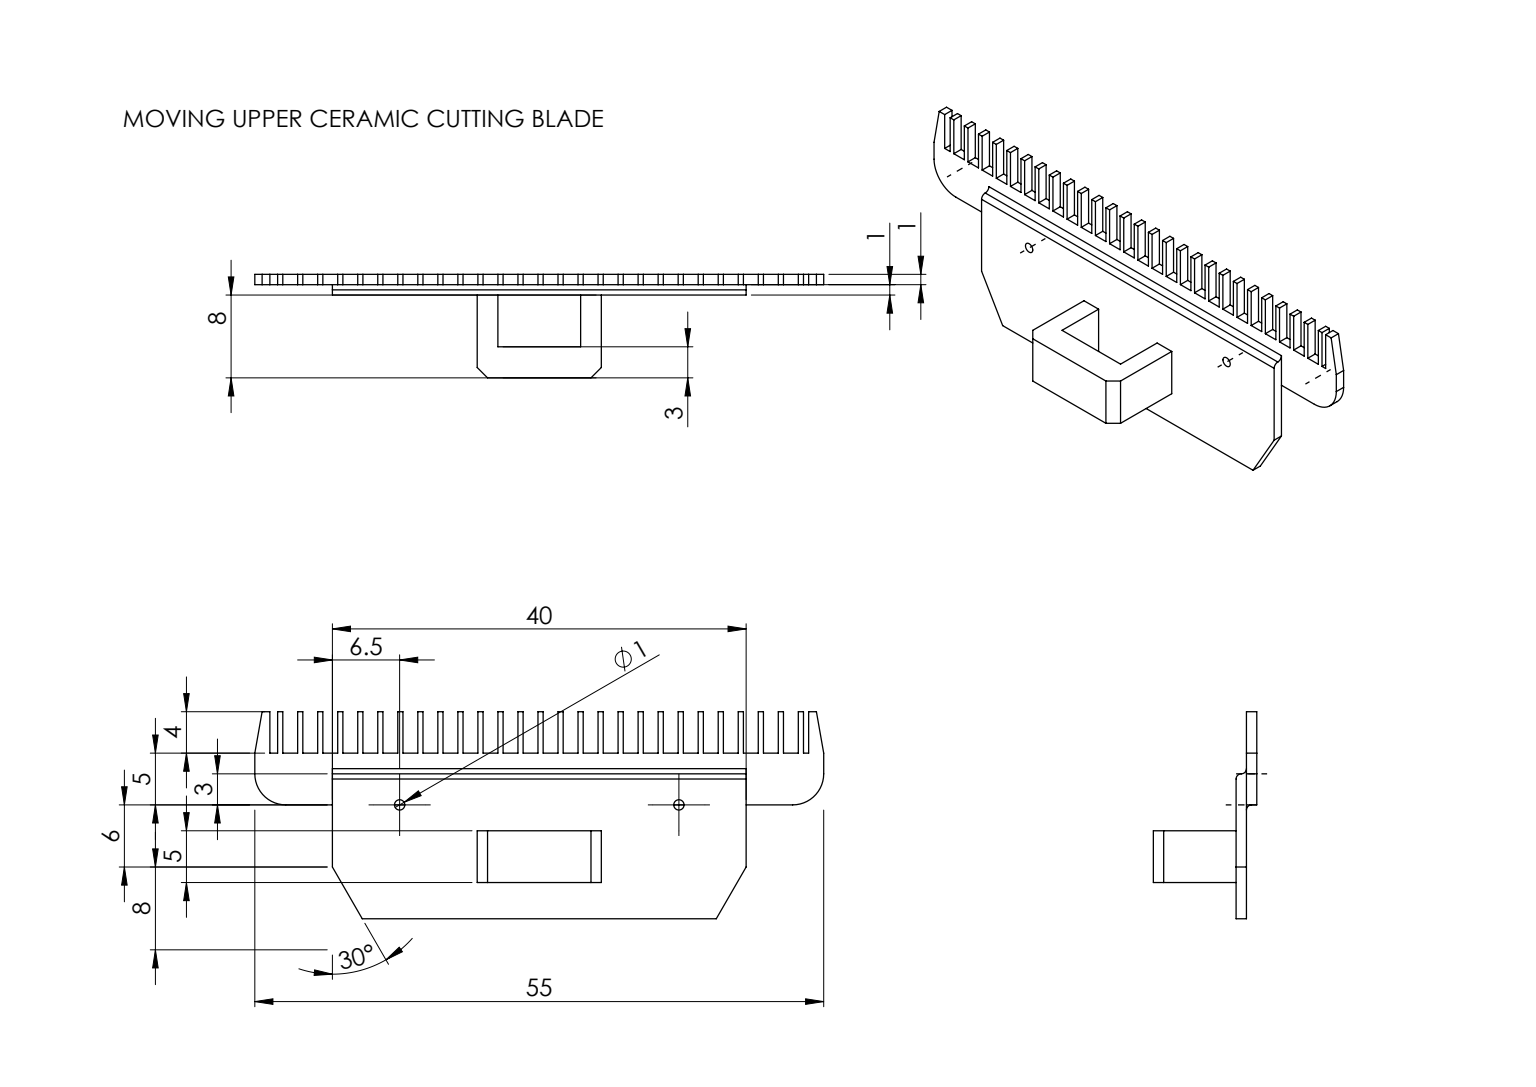
ISO-10303-21;
HEADER;
FILE_DESCRIPTION (('STEP AP214'),
    '1' );
FILE_NAME ('Moving Upper Ceramic Cutting Blade.step',
    '2026-10-04T16:38:04',
    ( '' ),
    ( '' ),
    'SwSTEP 2.0',
    'SolidWorks 2026',
    '' );
FILE_SCHEMA (( 'AUTOMOTIVE_DESIGN' ));
ENDSEC;

DATA;
#15=VECTOR ( 'NONE', #20550, 1000.000000000000000 ) ;
#17=VERTEX_POINT ( 'NONE', #19101 ) ;
#19=VERTEX_POINT ( 'NONE', #1418 ) ;
#21=FACE_BOUND ( 'NONE', #10951, .T. ) ;
#22=VECTOR ( 'NONE', #3512, 1000.000000000000000 ) ;
#26=FACE_OUTER_BOUND ( 'NONE', #4692, .T. ) ;
#35=ORIENTED_EDGE ( 'NONE', *, *, #2432, .F. ) ;
#42=VERTEX_POINT ( 'NONE', #6438 ) ;
#47=VECTOR ( 'NONE', #8617, 1000.000000000000000 ) ;
#49=VERTEX_POINT ( 'NONE', #11237 ) ;
#53=LINE ( 'NONE', #6129, #8350 ) ;
#54=AXIS2_PLACEMENT_3D ( 'NONE', #18555, #20450, #10501 ) ;
#56=LINE ( 'NONE', #9565, #7988 ) ;
#58=LINE ( 'NONE', #8001, #5190 ) ;
#60=CARTESIAN_POINT ( 'NONE',  ( 10.05565079891005631, 0.000000000000000000, 1.000000000000000000 ) ) ;
#61=LINE ( 'NONE', #4966, #6978 ) ;
#63=DIRECTION ( 'NONE',  ( 1.000000000000000000, 0.000000000000000000, 0.000000000000000000 ) ) ;
#68=VERTEX_POINT ( 'NONE', #1726 ) ;
#76=ORIENTED_EDGE ( 'NONE', *, *, #12428, .T. ) ;
#77=LINE ( 'NONE', #272, #14093 ) ;
#78=ORIENTED_EDGE ( 'NONE', *, *, #4872, .F. ) ;
#87=LINE ( 'NONE', #11371, #8961 ) ;
#89=( NAMED_UNIT ( * ) PLANE_ANGLE_UNIT ( ) SI_UNIT ( $, .RADIAN. ) );
#91=ORIENTED_EDGE ( 'NONE', *, *, #1253, .F. ) ;
#96=ADVANCED_FACE ( 'NONE', ( #6747 ), #14788, .T. ) ;
#98=DIRECTION ( 'NONE',  ( 0.000000000000000000, 1.000000000000000000, 0.000000000000000000 ) ) ;
#99=ORIENTED_EDGE ( 'NONE', *, *, #2749, .T. ) ;
#101=EDGE_LOOP ( 'NONE', ( #4164, #18704, #19121, #9760 ) ) ;
#102=VECTOR ( 'NONE', #3699, 1000.000000000000000 ) ;
#107=DIRECTION ( 'NONE',  ( -1.000000000000000000, 0.000000000000000000, 0.000000000000000000 ) ) ;
#114=VECTOR ( 'NONE', #15578, 1000.000000000000000 ) ;
#115=LINE ( 'NONE', #12457, #8728 ) ;
#121=ORIENTED_EDGE ( 'NONE', *, *, #545, .F. ) ;
#122=VERTEX_POINT ( 'NONE', #13311 ) ;
#126=ORIENTED_EDGE ( 'NONE', *, *, #7427, .F. ) ;
#128=CARTESIAN_POINT ( 'NONE',  ( 5.683390479346035029, 0.000000000000000000, 0.000000000000000000 ) ) ;
#134=CARTESIAN_POINT ( 'NONE',  ( -15.11404127825609223, 9.000000000000001776, 0.000000000000000000 ) ) ;
#137=LINE ( 'NONE', #12477, #19758 ) ;
#148=CARTESIAN_POINT ( 'NONE',  ( -24.79469207716615031, 9.000000000000001776, 1.000000000000000000 ) ) ;
#153=DIRECTION ( 'NONE',  ( 1.734723475976807094E-15, -1.000000000000000000, 0.000000000000000000 ) ) ;
#156=ORIENTED_EDGE ( 'NONE', *, *, #12533, .T. ) ;
#159=DIRECTION ( 'NONE',  ( 1.000000000000000000, 0.000000000000000000, 0.000000000000000000 ) ) ;
#161=CARTESIAN_POINT ( 'NONE',  ( 0.3749999999999968914, 9.000000000000000000, 1.000000000000000000 ) ) ;
#168=EDGE_LOOP ( 'NONE', ( #6512, #8849, #9507, #11718, #13942, #16405 ) ) ;
#170=DIRECTION ( 'NONE',  ( -0.000000000000000000, -0.000000000000000000, -1.000000000000000000 ) ) ;
#174=EDGE_CURVE ( 'NONE', #8535, #2052, #465, .T. ) ;
#177=ORIENTED_EDGE ( 'NONE', *, *, #14375, .F. ) ;
#179=FACE_OUTER_BOUND ( 'NONE', #19675, .T. ) ;
#180=AXIS2_PLACEMENT_3D ( 'NONE', #10679, #7642, #12344 ) ;
#187=LINE ( 'NONE', #10011, #17890 ) ;
#195=EDGE_CURVE ( 'NONE', #11770, #17871, #16650, .T. ) ;
#202=ORIENTED_EDGE ( 'NONE', *, *, #15005, .F. ) ;
#205=DIRECTION ( 'NONE',  ( 0.000000000000000000, -1.000000000000000000, 0.000000000000000000 ) ) ;
#208=DIRECTION ( 'NONE',  ( -0.9848077530122082424, 0.1736481776669295263, 0.000000000000000000 ) ) ;
#230=DIRECTION ( 'NONE',  ( -1.000000000000000000, -0.000000000000000000, -0.000000000000000000 ) ) ;
#231=CARTESIAN_POINT ( 'NONE',  ( 3.999999999999999112, -7.500000000000047073, 9.999999999999998224 ) ) ;
#259=EDGE_LOOP ( 'NONE', ( #9919, #6781, #19047, #17582 ) ) ;
#263=ORIENTED_EDGE ( 'NONE', *, *, #15990, .F. ) ;
#266=FACE_OUTER_BOUND ( 'NONE', #16647, .T. ) ;
#270=VECTOR ( 'NONE', #15636, 1000.000000000000000 ) ;
#272=CARTESIAN_POINT ( 'NONE',  ( 0.000000000000000000, 0.000000000000000000, 0.000000000000000000 ) ) ;
#274=ORIENTED_EDGE ( 'NONE', *, *, #17333, .T. ) ;
#278=LINE ( 'NONE', #14715, #12697 ) ;
#282=AXIS2_PLACEMENT_3D ( 'NONE', #5586, #11856, #17932 ) ;
#294=CARTESIAN_POINT ( 'NONE',  ( -3.497260319564023057, 9.000000000000001776, 0.000000000000000000 ) ) ;
#295=DIRECTION ( 'NONE',  ( 1.000000000000000000, 0.000000000000000000, 0.000000000000000000 ) ) ;
#302=VECTOR ( 'NONE', #7934, 1000.000000000000000 ) ;
#304=AXIS2_PLACEMENT_3D ( 'NONE', #2180, #611, #8776 ) ;
#305=ORIENTED_EDGE ( 'NONE', *, *, #7234, .F. ) ;
#306=VECTOR ( 'NONE', #18807, 1000.000000000000000 ) ;
#312=PLANE ( 'NONE',  #2667 ) ;
#324=ORIENTED_EDGE ( 'NONE', *, *, #17670, .T. ) ;
#325=ORIENTED_EDGE ( 'NONE', *, *, #12049, .T. ) ;
#328=CARTESIAN_POINT ( 'NONE',  ( 9.830951894845298966, -7.500000000000047073, 7.000000000000000000 ) ) ;
#331=EDGE_LOOP ( 'NONE', ( #16127, #14470, #13660, #8482 ) ) ;
#335=VECTOR ( 'NONE', #866, 1000.000000000000000 ) ;
#337=VECTOR ( 'NONE', #729, 1000.000000000000000 ) ;
#340=CARTESIAN_POINT ( 'NONE',  ( 0.000000000000000000, 4.999999999999999112, 1.000000000000000000 ) ) ;
#355=ORIENTED_EDGE ( 'NONE', *, *, #1510, .F. ) ;
#357=VECTOR ( 'NONE', #14447, 1000.000000000000000 ) ;
#358=ORIENTED_EDGE ( 'NONE', *, *, #6960, .T. ) ;
#360=CARTESIAN_POINT ( 'NONE',  ( 1.811130159782011528, 4.999999999999999112, 0.000000000000000000 ) ) ;
#366=CARTESIAN_POINT ( 'NONE',  ( 26.04469207716615031, 4.999999999999999112, 0.000000000000000000 ) ) ;
#367=VECTOR ( 'NONE', #7889, 1000.000000000000000 ) ;
#369=DIRECTION ( 'NONE',  ( -0.000000000000000000, 0.000000000000000000, -1.000000000000000000 ) ) ;
#370=DIRECTION ( 'NONE',  ( 0.000000000000000000, 1.000000000000000000, 0.000000000000000000 ) ) ;
#374=EDGE_LOOP ( 'NONE', ( #263, #11336, #20204, #3234 ) ) ;
#381=VERTEX_POINT ( 'NONE', #2855 ) ;
#385=ORIENTED_EDGE ( 'NONE', *, *, #8922, .T. ) ;
#404=DIRECTION ( 'NONE',  ( 1.000000000000000000, 0.000000000000000000, -0.000000000000000000 ) ) ;
#406=ORIENTED_EDGE ( 'NONE', *, *, #5858, .F. ) ;
#413=VECTOR ( 'NONE', #1830, 1000.000000000000000 ) ;
#416=DIRECTION ( 'NONE',  ( 0.000000000000000000, 1.000000000000000000, 0.000000000000000000 ) ) ;
#417=EDGE_CURVE ( 'NONE', #11328, #740, #20025, .T. ) ;
#427=VECTOR ( 'NONE', #3877, 1000.000000000000000 ) ;
#430=ORIENTED_EDGE ( 'NONE', *, *, #12679, .F. ) ;
#431=VERTEX_POINT ( 'NONE', #15503 ) ;
#435=ORIENTED_EDGE ( 'NONE', *, *, #9741, .F. ) ;
#448=EDGE_CURVE ( 'NONE', #18810, #17042, #19331, .T. ) ;
#457=CARTESIAN_POINT ( 'NONE',  ( -17.05017143803810242, 9.000000000000001776, 0.000000000000000000 ) ) ;
#458=VERTEX_POINT ( 'NONE', #10427 ) ;
#460=EDGE_LOOP ( 'NONE', ( #13036, #3328, #19557, #13078 ) ) ;
#463=DIRECTION ( 'NONE',  ( 0.000000000000000000, 1.000000000000000000, -0.000000000000000000 ) ) ;
#465=LINE ( 'NONE', #16554, #12981 ) ;
#469=LINE ( 'NONE', #14791, #1048 ) ;
#471=EDGE_CURVE ( 'NONE', #20320, #1300, #20347, .T. ) ;
#476=ORIENTED_EDGE ( 'NONE', *, *, #6440, .F. ) ;
#480=ORIENTED_EDGE ( 'NONE', *, *, #12324, .T. ) ;
#484=CARTESIAN_POINT ( 'NONE',  ( 0.000000000000000000, 9.000000000000001776, 1.000000000000000000 ) ) ;
#485=VERTEX_POINT ( 'NONE', #18066 ) ;
#487=VERTEX_POINT ( 'NONE', #8855 ) ;
#493=CARTESIAN_POINT ( 'NONE',  ( 3.999999999999999112, -2.500000000000047518, 7.000000000000000000 ) ) ;
#495=CARTESIAN_POINT ( 'NONE',  ( -11.24178095869206828, 0.000000000000000000, 1.000000000000000000 ) ) ;
#502=DIRECTION ( 'NONE',  ( -0.000000000000000000, -0.000000000000000000, -1.000000000000000000 ) ) ;
#504=ORIENTED_EDGE ( 'NONE', *, *, #11433, .F. ) ;
#506=ORIENTED_EDGE ( 'NONE', *, *, #871, .T. ) ;
#509=( GEOMETRIC_REPRESENTATION_CONTEXT ( 3 ) GLOBAL_UNCERTAINTY_ASSIGNED_CONTEXT ( ( #11112 ) ) GLOBAL_UNIT_ASSIGNED_CONTEXT ( ( #4790, #89, #18824 ) ) REPRESENTATION_CONTEXT ( 'NONE', 'WORKASPACE' ) );
#510=VERTEX_POINT ( 'NONE', #18268 ) ;
#511=DIRECTION ( 'NONE',  ( 0.000000000000000000, 1.000000000000000000, -0.000000000000000000 ) ) ;
#516=CARTESIAN_POINT ( 'NONE',  ( -13.50000000000000178, 0.000000000000000000, 2.000000000000000000 ) ) ;
#521=DIRECTION ( 'NONE',  ( 1.000000000000000000, 0.000000000000000000, 0.000000000000000000 ) ) ;
#537=SHAPE_REPRESENTATION ( 'Moving Upper Ceramic Cutting Blade', ( #18039 ), #19052 ) ;
#538=DIRECTION ( 'NONE',  ( -0.000000000000000000, -0.000000000000000000, -1.000000000000000000 ) ) ;
#543=CARTESIAN_POINT ( 'NONE',  ( -26.79469207716615387, 9.000000000000001776, 0.000000000000000000 ) ) ;
#545=EDGE_CURVE ( 'NONE', #15372, #1213, #2256, .T. ) ;
#548=VECTOR ( 'NONE', #15264, 1000.000000000000000 ) ;
#553=EDGE_CURVE ( 'NONE', #4594, #7048, #16384, .T. ) ;
#557=ORIENTED_EDGE ( 'NONE', *, *, #18497, .T. ) ;
#558=ORIENTED_EDGE ( 'NONE', *, *, #7385, .F. ) ;
#559=CARTESIAN_POINT ( 'NONE',  ( 24.50000000000000000, 3.000000000000000888, 1.000000000000000000 ) ) ;
#565=CARTESIAN_POINT ( 'NONE',  ( 11.99178095869207006, 9.000000000000001776, 1.000000000000000000 ) ) ;
#578=CARTESIAN_POINT ( 'NONE',  ( 1.811130159782011528, 0.000000000000000000, 1.000000000000000000 ) ) ;
#580=ORIENTED_EDGE ( 'NONE', *, *, #14379, .F. ) ;
#582=ORIENTED_EDGE ( 'NONE', *, *, #16071, .F. ) ;
#584=VECTOR ( 'NONE', #15881, 1000.000000000000000 ) ;
#591=ADVANCED_FACE ( 'NONE', ( #6870 ), #5194, .F. ) ;
#593=DIRECTION ( 'NONE',  ( 0.000000000000000000, 1.000000000000000000, -0.000000000000000000 ) ) ;
#605=ORIENTED_EDGE ( 'NONE', *, *, #19738, .F. ) ;
#607=VERTEX_POINT ( 'NONE', #11775 ) ;
#610=VERTEX_POINT ( 'NONE', #19851 ) ;
#611=DIRECTION ( 'NONE',  ( 1.000000000000000000, 0.000000000000000000, 0.000000000000000000 ) ) ;
#613=AXIS2_PLACEMENT_3D ( 'NONE', #19953, #11673, #2065 ) ;
#617=PLANE ( 'NONE',  #15078 ) ;
#618=CARTESIAN_POINT ( 'NONE',  ( 21.67243175760212637, 9.000000000000001776, 1.000000000000000000 ) ) ;
#622=FACE_OUTER_BOUND ( 'NONE', #5655, .T. ) ;
#627=CARTESIAN_POINT ( 'NONE',  ( 0.000000000000000000, 4.999999999999999112, 1.000000000000000000 ) ) ;
#632=CARTESIAN_POINT ( 'NONE',  ( -20.92243175760212637, 9.000000000000001776, 1.000000000000000000 ) ) ;
#633=ORIENTED_EDGE ( 'NONE', *, *, #1622, .T. ) ;
#640=CARTESIAN_POINT ( 'NONE',  ( -5.999999999999999112, -7.500000000000047073, 2.000000000000000000 ) ) ;
#643=LINE ( 'NONE', #752, #2713 ) ;
#646=CARTESIAN_POINT ( 'NONE',  ( 23.10856191738414012, 9.000000000000001776, 1.000000000000000000 ) ) ;
#652=ORIENTED_EDGE ( 'NONE', *, *, #14971, .T. ) ;
#656=AXIS2_PLACEMENT_3D ( 'NONE', #3159, #9531, #15903 ) ;
#657=ORIENTED_EDGE ( 'NONE', *, *, #3638, .T. ) ;
#661=EDGE_CURVE ( 'NONE', #485, #9583, #9261, .T. ) ;
#664=EDGE_CURVE ( 'NONE', #12892, #14133, #14065, .T. ) ;
#670=DIRECTION ( 'NONE',  ( 0.000000000000000000, 1.000000000000000000, -0.000000000000000000 ) ) ;
#671=DIRECTION ( 'NONE',  ( -1.000000000000000000, 0.000000000000000000, -0.000000000000000000 ) ) ;
#673=PLANE ( 'NONE',  #282 ) ;
#677=VECTOR ( 'NONE', #10798, 1000.000000000000000 ) ;
#684=DIRECTION ( 'NONE',  ( 0.000000000000000000, 1.000000000000000000, -0.000000000000000000 ) ) ;
#685=ORIENTED_EDGE ( 'NONE', *, *, #6597, .T. ) ;
#686=ORIENTED_EDGE ( 'NONE', *, *, #20030, .T. ) ;
#695=VECTOR ( 'NONE', #5802, 1000.000000000000000 ) ;
#702=PLANE ( 'NONE',  #15627 ) ;
#707=ORIENTED_EDGE ( 'NONE', *, *, #15426, .F. ) ;
#713=CARTESIAN_POINT ( 'NONE',  ( 27.52582389412042474, 4.853545418763153485, 0.000000000000000000 ) ) ;
#714=AXIS2_PLACEMENT_3D ( 'NONE', #5891, #15604, #12261 ) ;
#715=ORIENTED_EDGE ( 'NONE', *, *, #12942, .T. ) ;
#721=ORIENTED_EDGE ( 'NONE', *, *, #19909, .T. ) ;
#728=CARTESIAN_POINT ( 'NONE',  ( 0.000000000000000000, 4.999999999999999112, 0.000000000000000000 ) ) ;
#729=DIRECTION ( 'NONE',  ( 0.000000000000000000, 1.000000000000000000, -0.000000000000000000 ) ) ;
#732=EDGE_CURVE ( 'NONE', #15336, #11328, #16999, .T. ) ;
#734=VERTEX_POINT ( 'NONE', #2564 ) ;
#740=VERTEX_POINT ( 'NONE', #20055 ) ;
#744=ORIENTED_EDGE ( 'NONE', *, *, #16763, .T. ) ;
#746=CARTESIAN_POINT ( 'NONE',  ( 0.000000000000000000, 4.999999999999999112, 0.000000000000000000 ) ) ;
#747=DIRECTION ( 'NONE',  ( 0.000000000000000000, -0.000000000000000000, 1.000000000000000000 ) ) ;
#750=DIRECTION ( 'NONE',  ( 0.000000000000000000, 0.000000000000000000, 1.000000000000000000 ) ) ;
#752=CARTESIAN_POINT ( 'NONE',  ( -2.981555974335140152E-16, 2.500000000000002220, 2.000000000000000000 ) ) ;
#758=ADVANCED_FACE ( 'NONE', ( #4458 ), #15434, .T. ) ;
#759=LINE ( 'NONE', #1071, #677 ) ;
#769=DIRECTION ( 'NONE',  ( -0.000000000000000000, -0.000000000000000000, -1.000000000000000000 ) ) ;
#770=VECTOR ( 'NONE', #17153, 1000.000000000000000 ) ;
#775=DIRECTION ( 'NONE',  ( 0.000000000000000000, 0.000000000000000000, 1.000000000000000000 ) ) ;
#776=LINE ( 'NONE', #10288, #15723 ) ;
#778=CARTESIAN_POINT ( 'NONE',  ( -25.29469207716615031, 9.000000000000001776, 1.000000000000000000 ) ) ;
#781=ORIENTED_EDGE ( 'NONE', *, *, #10378, .T. ) ;
#791=ORIENTED_EDGE ( 'NONE', *, *, #13338, .F. ) ;
#792=LINE ( 'NONE', #7177, #1752 ) ;
#796=EDGE_CURVE ( 'NONE', #3716, #11889, #6025, .T. ) ;
#799=FACE_OUTER_BOUND ( 'NONE', #12254, .T. ) ;
#800=PLANE ( 'NONE',  #12000 ) ;
#801=DIRECTION ( 'NONE',  ( 0.000000000000000000, 0.000000000000000000, 1.000000000000000000 ) ) ;
#807=CARTESIAN_POINT ( 'NONE',  ( -13.67791111847408025, 4.999999999999999112, 0.000000000000000000 ) ) ;
#811=ORIENTED_EDGE ( 'NONE', *, *, #14623, .T. ) ;
#816=DIRECTION ( 'NONE',  ( -0.000000000000000000, 0.000000000000000000, -1.000000000000000000 ) ) ;
#819=ORIENTED_EDGE ( 'NONE', *, *, #12042, .F. ) ;
#820=ORIENTED_EDGE ( 'NONE', *, *, #2735, .F. ) ;
#821=EDGE_CURVE ( 'NONE', #7330, #19819, #20258, .T. ) ;
#825=DIRECTION ( 'NONE',  ( 1.000000000000000000, 0.000000000000000000, -0.000000000000000000 ) ) ;
#826=CARTESIAN_POINT ( 'NONE',  ( 2.311130159782011972, 4.999999999999999112, 0.000000000000000000 ) ) ;
#827=CARTESIAN_POINT ( 'NONE',  ( -11.24178095869206828, 9.000000000000001776, 1.000000000000000000 ) ) ;
#843=DIRECTION ( 'NONE',  ( 0.000000000000000000, 1.000000000000000000, 0.000000000000000000 ) ) ;
#845=ORIENTED_EDGE ( 'NONE', *, *, #9874, .T. ) ;
#847=DIRECTION ( 'NONE',  ( -0.000000000000000000, -0.000000000000000000, -1.000000000000000000 ) ) ;
#848=DIRECTION ( 'NONE',  ( 1.000000000000000000, 0.000000000000000000, 0.000000000000000000 ) ) ;
#854=FACE_OUTER_BOUND ( 'NONE', #19395, .T. ) ;
#866=DIRECTION ( 'NONE',  ( 0.000000000000000000, -0.000000000000000000, 1.000000000000000000 ) ) ;
#869=CARTESIAN_POINT ( 'NONE',  ( 10.05565079891005631, 4.999999999999999112, 1.000000000000000000 ) ) ;
#870=VECTOR ( 'NONE', #16492, 1000.000000000000000 ) ;
#871=EDGE_CURVE ( 'NONE', #1300, #20320, #11999, .T. ) ;
#889=ORIENTED_EDGE ( 'NONE', *, *, #6722, .T. ) ;
#892=ORIENTED_EDGE ( 'NONE', *, *, #4514, .T. ) ;
#894=ORIENTED_EDGE ( 'NONE', *, *, #18955, .F. ) ;
#895=CARTESIAN_POINT ( 'NONE',  ( -17.05017143803810242, 9.000000000000001776, 1.000000000000000000 ) ) ;
#908=ORIENTED_EDGE ( 'NONE', *, *, #5009, .T. ) ;
#912=LINE ( 'NONE', #5519, #930 ) ;
#918=DIRECTION ( 'NONE',  ( 0.000000000000000000, -0.000000000000000000, 1.000000000000000000 ) ) ;
#919=FACE_OUTER_BOUND ( 'NONE', #16776, .T. ) ;
#924=VECTOR ( 'NONE', #1979, 1000.000000000000000 ) ;
#925=LINE ( 'NONE', #827, #16027 ) ;
#927=EDGE_CURVE ( 'NONE', #15982, #12948, #56, .T. ) ;
#930=VECTOR ( 'NONE', #4368, 1000.000000000000000 ) ;
#936=EDGE_CURVE ( 'NONE', #17, #20705, #15840, .T. ) ;
#940=ORIENTED_EDGE ( 'NONE', *, *, #4469, .F. ) ;
#942=DIRECTION ( 'NONE',  ( -0.000000000000000000, -0.000000000000000000, -1.000000000000000000 ) ) ;
#943=ORIENTED_EDGE ( 'NONE', *, *, #17591, .T. ) ;
#944=AXIS2_PLACEMENT_3D ( 'NONE', #2419, #18922, #9187 ) ;
#945=CARTESIAN_POINT ( 'NONE',  ( 9.555650798910054533, 0.000000000000000000, 1.000000000000000000 ) ) ;
#946=DIRECTION ( 'NONE',  ( -0.000000000000000000, -0.000000000000000000, -1.000000000000000000 ) ) ;
#954=CARTESIAN_POINT ( 'NONE',  ( 9.555650798910054533, 9.000000000000001776, 1.000000000000000000 ) ) ;
#956=AXIS2_PLACEMENT_3D ( 'NONE', #10190, #19720, #5172 ) ;
#959=EDGE_CURVE ( 'NONE', #17043, #11462, #15938, .T. ) ;
#969=DIRECTION ( 'NONE',  ( 1.000000000000000000, 0.000000000000000000, -0.000000000000000000 ) ) ;
#970=EDGE_CURVE ( 'NONE', #122, #20224, #19412, .T. ) ;
#971=VECTOR ( 'NONE', #5445, 1000.000000000000000 ) ;
#980=LINE ( 'NONE', #17184, #6298 ) ;
#983=AXIS2_PLACEMENT_3D ( 'NONE', #16894, #20474, #12499 ) ;
#984=ORIENTED_EDGE ( 'NONE', *, *, #7515, .F. ) ;
#997=EDGE_LOOP ( 'NONE', ( #14226, #5207, #13822, #2454 ) ) ;
#999=VERTEX_POINT ( 'NONE', #14478 ) ;
#1005=LINE ( 'NONE', #7699, #8827 ) ;
#1010=DIRECTION ( 'NONE',  ( -1.000000000000000000, -1.192622389734054877E-16, 0.000000000000000000 ) ) ;
#1020=VECTOR ( 'NONE', #18657, 1000.000000000000000 ) ;
#1021=VECTOR ( 'NONE', #20699, 1000.000000000000000 ) ;
#1028=VECTOR ( 'NONE', #4358, 1000.000000000000000 ) ;
#1029=VECTOR ( 'NONE', #5552, 1000.000000000000000 ) ;
#1037=CARTESIAN_POINT ( 'NONE',  ( 3.747260319564023501, 0.000000000000000000, 0.000000000000000000 ) ) ;
#1040=VECTOR ( 'NONE', #11032, 1000.000000000000000 ) ;
#1048=VECTOR ( 'NONE', #18245, 1000.000000000000000 ) ;
#1051=CARTESIAN_POINT ( 'NONE',  ( 4.247260319564023945, 0.000000000000000000, 1.000000000000000000 ) ) ;
#1052=ORIENTED_EDGE ( 'NONE', *, *, #10950, .F. ) ;
#1053=ORIENTED_EDGE ( 'NONE', *, *, #3524, .T. ) ;
#1058=FACE_OUTER_BOUND ( 'NONE', #15885, .T. ) ;
#1061=ORIENTED_EDGE ( 'NONE', *, *, #19045, .T. ) ;
#1065=CARTESIAN_POINT ( 'NONE',  ( 11.99178095869207006, 9.000000000000001776, 0.000000000000000000 ) ) ;
#1071=CARTESIAN_POINT ( 'NONE',  ( -1.561130159782011306, 9.000000000000001776, 1.000000000000000000 ) ) ;
#1074=EDGE_CURVE ( 'NONE', #10713, #19625, #10285, .T. ) ;
#1080=ORIENTED_EDGE ( 'NONE', *, *, #1425, .F. ) ;
#1081=UNCERTAINTY_MEASURE_WITH_UNIT (LENGTH_MEASURE( 1.000000000000000082E-05 ), #17353, 'distance_accuracy_value', 'NONE');
#1082=ORIENTED_EDGE ( 'NONE', *, *, #7355, .F. ) ;
#1083=DIRECTION ( 'NONE',  ( 0.000000000000000000, -1.000000000000000000, 0.000000000000000000 ) ) ;
#1092=FACE_OUTER_BOUND ( 'NONE', #7198, .T. ) ;
#1105=DIRECTION ( 'NONE',  ( 1.000000000000000000, 0.000000000000000000, -0.000000000000000000 ) ) ;
#1109=DIRECTION ( 'NONE',  ( 0.000000000000000000, 1.000000000000000000, 0.000000000000000000 ) ) ;
#1111=VERTEX_POINT ( 'NONE', #3595 ) ;
#1113=DIRECTION ( 'NONE',  ( 0.000000000000000000, -1.000000000000000000, 0.000000000000000000 ) ) ;
#1114=ORIENTED_EDGE ( 'NONE', *, *, #4469, .T. ) ;
#1115=CARTESIAN_POINT ( 'NONE',  ( -22.85856191738413656, 4.999999999999999112, 1.000000000000000000 ) ) ;
#1117=LINE ( 'NONE', #18579, #5327 ) ;
#1125=LINE ( 'NONE', #17006, #6012 ) ;
#1134=FACE_OUTER_BOUND ( 'NONE', #3521, .T. ) ;
#1137=VERTEX_POINT ( 'NONE', #1925 ) ;
#1142=CARTESIAN_POINT ( 'NONE',  ( -5.999999999999999112, -7.500000000000047073, 9.999999999999998224 ) ) ;
#1145=VECTOR ( 'NONE', #205, 1000.000000000000000 ) ;
#1149=VERTEX_POINT ( 'NONE', #11547 ) ;
#1154=FACE_OUTER_BOUND ( 'NONE', #17723, .T. ) ;
#1161=ORIENTED_EDGE ( 'NONE', *, *, #12049, .F. ) ;
#1164=CARTESIAN_POINT ( 'NONE',  ( 0.000000000000000000, 0.000000000000000000, 1.000000000000000000 ) ) ;
#1166=EDGE_CURVE ( 'NONE', #9041, #10510, #13117, .T. ) ;
#1171=CARTESIAN_POINT ( 'NONE',  ( 19.23630159782011617, 4.999999999999999112, 1.000000000000000000 ) ) ;
#1181=ORIENTED_EDGE ( 'NONE', *, *, #2244, .T. ) ;
#1182=CARTESIAN_POINT ( 'NONE',  ( 6.183390479346035917, 9.000000000000001776, 0.000000000000000000 ) ) ;
#1184=VECTOR ( 'NONE', #2415, 1000.000000000000000 ) ;
#1196=EDGE_LOOP ( 'NONE', ( #1515, #11815, #721, #16544 ) ) ;
#1208=ORIENTED_EDGE ( 'NONE', *, *, #4382, .T. ) ;
#1209=LINE ( 'NONE', #13947, #18796 ) ;
#1213=VERTEX_POINT ( 'NONE', #11750 ) ;
#1220=LINE ( 'NONE', #7595, #4069 ) ;
#1221=DIRECTION ( 'NONE',  ( 0.000000000000000000, -0.000000000000000000, 1.000000000000000000 ) ) ;
#1222=DIRECTION ( 'NONE',  ( -0.000000000000000000, -0.000000000000000000, -1.000000000000000000 ) ) ;
#1223=DIRECTION ( 'NONE',  ( -0.000000000000000000, -0.000000000000000000, -1.000000000000000000 ) ) ;
#1228=EDGE_LOOP ( 'NONE', ( #5307, #10202, #12279, #10206 ) ) ;
#1236=ORIENTED_EDGE ( 'NONE', *, *, #17024, .T. ) ;
#1237=DIRECTION ( 'NONE',  ( -0.000000000000000000, 0.000000000000000000, 1.000000000000000000 ) ) ;
#1247=SURFACE_STYLE_USAGE ( .BOTH. , #7732 ) ;
#1251=LINE ( 'NONE', #7738, #13752 ) ;
#1253=EDGE_CURVE ( 'NONE', #8718, #122, #12062, .T. ) ;
#1256=EDGE_LOOP ( 'NONE', ( #18237, #3582, #15612, #20012 ) ) ;
#1257=ORIENTED_EDGE ( 'NONE', *, *, #16437, .T. ) ;
#1259=DIRECTION ( 'NONE',  ( 1.000000000000000000, 1.013672804646636068E-16, 0.000000000000000000 ) ) ;
#1260=FILL_AREA_STYLE ('',( #15784 ) ) ;
#1272=DIRECTION ( 'NONE',  ( 0.000000000000000000, -1.000000000000000000, 0.000000000000000000 ) ) ;
#1279=ORIENTED_EDGE ( 'NONE', *, *, #936, .T. ) ;
#1288=CARTESIAN_POINT ( 'NONE',  ( 10.05565079891005631, 4.999999999999999112, 0.000000000000000000 ) ) ;
#1290=CARTESIAN_POINT ( 'NONE',  ( 14.00000000000000000, 7.867487981852999499E-15, 2.000000000000000000 ) ) ;
#1300=VERTEX_POINT ( 'NONE', #10814 ) ;
#1309=VECTOR ( 'NONE', #3879, 1000.000000000000000 ) ;
#1315=VERTEX_POINT ( 'NONE', #7668 ) ;
#1318=DIRECTION ( 'NONE',  ( -0.000000000000000000, -0.000000000000000000, -1.000000000000000000 ) ) ;
#1328=PRODUCT_DEFINITION_SHAPE ( 'NONE', 'NONE',  #13790 ) ;
#1333=EDGE_LOOP ( 'NONE', ( #7064, #9377, #7104, #5763 ) ) ;
#1336=EDGE_LOOP ( 'NONE', ( #16230, #11844, #20016, #16927 ) ) ;
#1341=VECTOR ( 'NONE', #9743, 1000.000000000000000 ) ;
#1343=DIRECTION ( 'NONE',  ( 1.000000000000000000, 0.000000000000000000, 0.000000000000000000 ) ) ;
#1344=FACE_OUTER_BOUND ( 'NONE', #5696, .T. ) ;
#1345=VECTOR ( 'NONE', #17736, 1000.000000000000114 ) ;
#1347=PLANE ( 'NONE',  #2016 ) ;
#1348=DIRECTION ( 'NONE',  ( 0.000000000000000000, 1.000000000000000000, -0.000000000000000000 ) ) ;
#1349=DIRECTION ( 'NONE',  ( 0.000000000000000000, 0.000000000000000000, 1.000000000000000000 ) ) ;
#1353=ORIENTED_EDGE ( 'NONE', *, *, #7385, .T. ) ;
#1355=DIRECTION ( 'NONE',  ( -0.000000000000000000, -0.000000000000000000, -1.000000000000000000 ) ) ;
#1361=FACE_OUTER_BOUND ( 'NONE', #2818, .T. ) ;
#1363=VERTEX_POINT ( 'NONE', #7566 ) ;
#1371=LINE ( 'NONE', #20620, #5508 ) ;
#1388=AXIS2_PLACEMENT_3D ( 'NONE', #14457, #15917, #6202 ) ;
#1391=DIRECTION ( 'NONE',  ( 0.000000000000000000, 0.000000000000000000, -1.000000000000000000 ) ) ;
#1394=EDGE_CURVE ( 'NONE', #5367, #10647, #4116, .T. ) ;
#1400=VECTOR ( 'NONE', #15536, 1000.000000000000000 ) ;
#1417=CARTESIAN_POINT ( 'NONE',  ( -13.82942202582513325, -0.3863038687793825532, 0.9889833525439024609 ) ) ;
#1418=CARTESIAN_POINT ( 'NONE',  ( 17.30017143803810242, 4.999999999999999112, 1.000000000000000000 ) ) ;
#1420=LINE ( 'NONE', #7695, #9692 ) ;
#1423=CARTESIAN_POINT ( 'NONE',  ( 11.49178095869207006, 0.000000000000000000, 1.000000000000000000 ) ) ;
#1425=EDGE_CURVE ( 'NONE', #10713, #6994, #6105, .T. ) ;
#1426=CARTESIAN_POINT ( 'NONE',  ( 0.000000000000000000, 9.000000000000001776, 0.000000000000000000 ) ) ;
#1438=ORIENTED_EDGE ( 'NONE', *, *, #20290, .F. ) ;
#1446=DIRECTION ( 'NONE',  ( -0.000000000000000000, -0.000000000000000000, -1.000000000000000000 ) ) ;
#1448=DIRECTION ( 'NONE',  ( 0.000000000000000000, 1.000000000000000000, 0.000000000000000000 ) ) ;
#1449=CARTESIAN_POINT ( 'NONE',  ( -7.869520639128047002, 0.000000000000000000, 0.000000000000000000 ) ) ;
#1450=ADVANCED_FACE ( 'NONE', ( #13828 ), #9233, .T. ) ;
#1451=DIRECTION ( 'NONE',  ( 0.000000000000000000, 1.000000000000000000, 0.000000000000000000 ) ) ;
#1456=CARTESIAN_POINT ( 'NONE',  ( -25.29469207716615031, 4.999999999999999112, 1.000000000000000000 ) ) ;
#1458=VERTEX_POINT ( 'NONE', #1288 ) ;
#1469=FACE_OUTER_BOUND ( 'NONE', #6490, .T. ) ;
#1486=EDGE_CURVE ( 'NONE', #19789, #8535, #7778, .T. ) ;
#1488=LINE ( 'NONE', #1796, #11778 ) ;
#1491=DIRECTION ( 'NONE',  ( -0.000000000000000000, 0.000000000000000000, -1.000000000000000000 ) ) ;
#1496=CARTESIAN_POINT ( 'NONE',  ( 5.999999999999999112, -7.500000000000047073, 2.000000000000000000 ) ) ;
#1509=EDGE_LOOP ( 'NONE', ( #2058, #14157, #12109, #10635 ) ) ;
#1510=EDGE_CURVE ( 'NONE', #10510, #9451, #4528, .T. ) ;
#1511=EDGE_LOOP ( 'NONE', ( #9435, #10300, #10130, #6368 ) ) ;
#1513=AXIS2_PLACEMENT_3D ( 'NONE', #3783, #7028, #19050 ) ;
#1515=ORIENTED_EDGE ( 'NONE', *, *, #6636, .F. ) ;
#1521=DIRECTION ( 'NONE',  ( 0.000000000000000000, -0.000000000000000000, 1.000000000000000000 ) ) ;
#1523=DIRECTION ( 'NONE',  ( -1.000000000000000000, -1.192622389734054877E-16, 0.000000000000000000 ) ) ;
#1526=MECHANICAL_DESIGN_GEOMETRIC_PRESENTATION_REPRESENTATION('',(#14541),#509);
#1531=ORIENTED_EDGE ( 'NONE', *, *, #8139, .T. ) ;
#1537=DIRECTION ( 'NONE',  ( -1.000000000000000000, 0.000000000000000000, 0.000000000000000000 ) ) ;
#1539=VECTOR ( 'NONE', #5300, 1000.000000000000000 ) ;
#1540=ORIENTED_EDGE ( 'NONE', *, *, #16503, .F. ) ;
#1541=DIRECTION ( 'NONE',  ( 1.000000000000000000, 0.000000000000000000, 0.000000000000000000 ) ) ;
#1544=LINE ( 'NONE', #4680, #1021 ) ;
#1551=LINE ( 'NONE', #19243, #17083 ) ;
#1558=LINE ( 'NONE', #1666, #5256 ) ;
#1560=EDGE_CURVE ( 'NONE', #16909, #8663, #1704, .T. ) ;
#1580=ORIENTED_EDGE ( 'NONE', *, *, #11475, .T. ) ;
#1583=VERTEX_POINT ( 'NONE', #134 ) ;
#1586=LINE ( 'NONE', #4830, #2775 ) ;
#1613=DIRECTION ( 'NONE',  ( 1.000000000000000000, 0.000000000000000000, 0.000000000000000000 ) ) ;
#1621=CARTESIAN_POINT ( 'NONE',  ( -5.999999999999999112, -7.500000000000047073, 9.999999999999998224 ) ) ;
#1622=EDGE_CURVE ( 'NONE', #11456, #10835, #3473, .T. ) ;
#1623=DIRECTION ( 'NONE',  ( 0.000000000000000000, -1.000000000000000000, 0.000000000000000000 ) ) ;
#1624=DIRECTION ( 'NONE',  ( -0.000000000000000000, -0.000000000000000000, -1.000000000000000000 ) ) ;
#1636=VERTEX_POINT ( 'NONE', #8285 ) ;
#1641=ORIENTED_EDGE ( 'NONE', *, *, #13351, .F. ) ;
#1645=ORIENTED_EDGE ( 'NONE', *, *, #19492, .T. ) ;
#1656=ORIENTED_EDGE ( 'NONE', *, *, #17797, .T. ) ;
#1662=LINE ( 'NONE', #17771, #14658 ) ;
#1666=CARTESIAN_POINT ( 'NONE',  ( -13.67791111847408025, 9.000000000000001776, 1.000000000000000000 ) ) ;
#1670=ORIENTED_EDGE ( 'NONE', *, *, #1949, .F. ) ;
#1673=CARTESIAN_POINT ( 'NONE',  ( 24.50000000000000000, 3.000000000000000888, 0.000000000000000000 ) ) ;
#1681=AXIS2_PLACEMENT_3D ( 'NONE', #12774, #4831, #3568 ) ;
#1688=VERTEX_POINT ( 'NONE', #3572 ) ;
#1690=EDGE_CURVE ( 'NONE', #14252, #14385, #643, .T. ) ;
#1692=ADVANCED_FACE ( 'NONE', ( #18220 ), #6822, .T. ) ;
#1693=CARTESIAN_POINT ( 'NONE',  ( -22.85856191738413656, 4.999999999999999112, 1.000000000000000000 ) ) ;
#1696=PRODUCT_DEFINITION_FORMATION_WITH_SPECIFIED_SOURCE ( 'ANY', '', #6339, .NOT_KNOWN. ) ;
#1697=ORIENTED_EDGE ( 'NONE', *, *, #12211, .F. ) ;
#1701=FACE_OUTER_BOUND ( 'NONE', #10294, .T. ) ;
#1704=LINE ( 'NONE', #8188, #12056 ) ;
#1706=LINE ( 'NONE', #16030, #3419 ) ;
#1707=DIRECTION ( 'NONE',  ( 1.000000000000000000, 0.000000000000000000, 0.000000000000000000 ) ) ;
#1711=ORIENTED_EDGE ( 'NONE', *, *, #2479, .F. ) ;
#1714=VECTOR ( 'NONE', #10709, 1000.000000000000000 ) ;
#1717=ORIENTED_EDGE ( 'NONE', *, *, #4886, .T. ) ;
#1721=DIRECTION ( 'NONE',  ( -1.000000000000000000, 0.000000000000000000, 0.000000000000000000 ) ) ;
#1726=CARTESIAN_POINT ( 'NONE',  ( -26.04469207716615031, 9.000000000000001776, 0.000000000000000000 ) ) ;
#1727=AXIS2_PLACEMENT_3D ( 'NONE', #17344, #1355, #11272 ) ;
#1746=ORIENTED_EDGE ( 'NONE', *, *, #2905, .F. ) ;
#1748=LINE ( 'NONE', #19628, #2042 ) ;
#1750=CARTESIAN_POINT ( 'NONE',  ( 5.683390479346035029, 4.999999999999999112, 1.000000000000000000 ) ) ;
#1751=ORIENTED_EDGE ( 'NONE', *, *, #17024, .F. ) ;
#1752=VECTOR ( 'NONE', #18473, 1000.000000000000000 ) ;
#1758=VECTOR ( 'NONE', #11337, 1000.000000000000000 ) ;
#1760=FACE_OUTER_BOUND ( 'NONE', #11634, .T. ) ;
#1762=ORIENTED_EDGE ( 'NONE', *, *, #7611, .F. ) ;
#1768=CARTESIAN_POINT ( 'NONE',  ( 9.555650798910054533, 0.000000000000000000, 0.000000000000000000 ) ) ;
#1769=ORIENTED_EDGE ( 'NONE', *, *, #19488, .F. ) ;
#1773=LINE ( 'NONE', #17248, #15470 ) ;
#1774=ORIENTED_EDGE ( 'NONE', *, *, #5845, .F. ) ;
#1780=CARTESIAN_POINT ( 'NONE',  ( -23.35856191738413656, 4.999999999999999112, 0.000000000000000000 ) ) ;
#1793=CARTESIAN_POINT ( 'NONE',  ( 0.000000000000000000, 0.000000000000000000, 0.000000000000000000 ) ) ;
#1794=ORIENTED_EDGE ( 'NONE', *, *, #2779, .F. ) ;
#1796=CARTESIAN_POINT ( 'NONE',  ( -19.48630159782011262, 9.000000000000001776, 1.000000000000000000 ) ) ;
#1798=EDGE_CURVE ( 'NONE', #15962, #4449, #8495, .T. ) ;
#1802=EDGE_CURVE ( 'NONE', #1213, #6097, #2210, .T. ) ;
#1805=DIRECTION ( 'NONE',  ( -0.000000000000000000, -0.000000000000000000, -1.000000000000000000 ) ) ;
#1815=ORIENTED_EDGE ( 'NONE', *, *, #1074, .F. ) ;
#1818=LINE ( 'NONE', #17918, #2993 ) ;
#1821=DIRECTION ( 'NONE',  ( -1.000000000000000000, 0.000000000000000000, 0.000000000000000000 ) ) ;
#1822=EDGE_CURVE ( 'NONE', #16179, #9059, #11423, .T. ) ;
#1830=DIRECTION ( 'NONE',  ( 1.000000000000000000, 0.000000000000000000, 0.000000000000000000 ) ) ;
#1831=LINE ( 'NONE', #161, #18030 ) ;
#1842=VECTOR ( 'NONE', #7752, 1000.000000000000000 ) ;
#1843=DIRECTION ( 'NONE',  ( -1.000000000000000000, -1.192622389734054877E-16, 0.000000000000000000 ) ) ;
#1844=VERTEX_POINT ( 'NONE', #15484 ) ;
#1850=AXIS2_PLACEMENT_3D ( 'NONE', #20670, #3289, #19308 ) ;
#1867=LINE ( 'NONE', #16401, #20324 ) ;
#1874=EDGE_CURVE ( 'NONE', #11254, #11965, #7546, .T. ) ;
#1875=ORIENTED_EDGE ( 'NONE', *, *, #10161, .F. ) ;
#1879=AXIS2_PLACEMENT_3D ( 'NONE', #7536, #2829, #7437 ) ;
#1892=ORIENTED_EDGE ( 'NONE', *, *, #6039, .T. ) ;
#1896=ORIENTED_EDGE ( 'NONE', *, *, #3165, .T. ) ;
#1897=ORIENTED_EDGE ( 'NONE', *, *, #3339, .T. ) ;
#1909=ORIENTED_EDGE ( 'NONE', *, *, #15811, .T. ) ;
#1913=EDGE_CURVE ( 'NONE', #740, #4847, #10793, .T. ) ;
#1916=ORIENTED_EDGE ( 'NONE', *, *, #8465, .F. ) ;
#1925=CARTESIAN_POINT ( 'NONE',  ( 1.811130159782011528, 9.000000000000001776, 1.000000000000000000 ) ) ;
#1928=CARTESIAN_POINT ( 'NONE',  ( 0.3749999999999968914, 9.000000000000000000, 1.000000000000000000 ) ) ;
#1931=DIRECTION ( 'NONE',  ( -0.000000000000000000, -0.000000000000000000, -1.000000000000000000 ) ) ;
#1934=ORIENTED_EDGE ( 'NONE', *, *, #19670, .T. ) ;
#1937=EDGE_CURVE ( 'NONE', #14589, #15962, #18431, .T. ) ;
#1943=ORIENTED_EDGE ( 'NONE', *, *, #17724, .F. ) ;
#1946=ORIENTED_EDGE ( 'NONE', *, *, #12802, .F. ) ;
#1949=EDGE_CURVE ( 'NONE', #12873, #1137, #9012, .T. ) ;
#1957=VECTOR ( 'NONE', #11825, 1000.000000000000000 ) ;
#1968=CARTESIAN_POINT ( 'NONE',  ( -20.00000000000000000, 3.499999999999999556, 1.500000000000000000 ) ) ;
#1971=VECTOR ( 'NONE', #1318, 1000.000000000000000 ) ;
#1973=ORIENTED_EDGE ( 'NONE', *, *, #18654, .F. ) ;
#1979=DIRECTION ( 'NONE',  ( -0.000000000000000000, -0.000000000000000000, -1.000000000000000000 ) ) ;
#1982=DIRECTION ( 'NONE',  ( -0.000000000000000000, -0.000000000000000000, -1.000000000000000000 ) ) ;
#1988=EDGE_CURVE ( 'NONE', #15008, #14162, #18744, .T. ) ;
#1991=DIRECTION ( 'NONE',  ( 1.000000000000000000, 0.000000000000000000, 0.000000000000000000 ) ) ;
#2000=DIRECTION ( 'NONE',  ( -0.000000000000000000, -0.000000000000000000, -1.000000000000000000 ) ) ;
#2001=VECTOR ( 'NONE', #4648, 1000.000000000000000 ) ;
#2002=PLANE ( 'NONE',  #13039 ) ;
#2005=STYLED_ITEM ( 'NONE', ( #4286 ), #15532 ) ;
#2016=AXIS2_PLACEMENT_3D ( 'NONE', #7727, #17954, #8239 ) ;
#2020=VERTEX_POINT ( 'NONE', #16848 ) ;
#2023=CARTESIAN_POINT ( 'NONE',  ( 0.000000000000000000, 4.999999999999999112, 0.000000000000000000 ) ) ;
#2024=ORIENTED_EDGE ( 'NONE', *, *, #17592, .T. ) ;
#2025=VECTOR ( 'NONE', #946, 1000.000000000000000 ) ;
#2026=EDGE_LOOP ( 'NONE', ( #6998, #5862, #6381, #5854 ) ) ;
#2027=CARTESIAN_POINT ( 'NONE',  ( -4.999999999999998224, 0.000000000000000000, 9.999999999999998224 ) ) ;
#2028=ADVANCED_FACE ( 'NONE', ( #9519 ), #15997, .T. ) ;
#2034=VECTOR ( 'NONE', #3246, 1000.000000000000000 ) ;
#2035=CARTESIAN_POINT ( 'NONE',  ( 20.00000000000000000, -5.999999999999994671, 2.000000000000000000 ) ) ;
#2041=VECTOR ( 'NONE', #4095, 1000.000000000000000 ) ;
#2042=VECTOR ( 'NONE', #5090, 1000.000000000000000 ) ;
#2051=CARTESIAN_POINT ( 'NONE',  ( 8.119520639128047890, 9.000000000000001776, 0.000000000000000000 ) ) ;
#2052=VERTEX_POINT ( 'NONE', #4816 ) ;
#2058=ORIENTED_EDGE ( 'NONE', *, *, #18139, .F. ) ;
#2063=LINE ( 'NONE', #18067, #12664 ) ;
#2065=DIRECTION ( 'NONE',  ( 0.000000000000000000, -0.000000000000000000, 1.000000000000000000 ) ) ;
#2072=VERTEX_POINT ( 'NONE', #9424 ) ;
#2075=VERTEX_POINT ( 'NONE', #14428 ) ;
#2076=DIRECTION ( 'NONE',  ( -1.000000000000000000, 0.000000000000000000, 0.000000000000000000 ) ) ;
#2080=ORIENTED_EDGE ( 'NONE', *, *, #9533, .T. ) ;
#2083=CARTESIAN_POINT ( 'NONE',  ( 15.86404127825609400, 4.999999999999999112, 1.000000000000000000 ) ) ;
#2085=DIRECTION ( 'NONE',  ( 1.000000000000000000, 0.000000000000000000, 0.000000000000000000 ) ) ;
#2091=VECTOR ( 'NONE', #8690, 1000.000000000000000 ) ;
#2096=VECTOR ( 'NONE', #14954, 1000.000000000000000 ) ;
#2103=ORIENTED_EDGE ( 'NONE', *, *, #19635, .T. ) ;
#2105=DIRECTION ( 'NONE',  ( 0.000000000000000000, -1.000000000000000000, 0.000000000000000000 ) ) ;
#2106=CARTESIAN_POINT ( 'NONE',  ( -9.305650798910056309, 9.000000000000001776, 0.000000000000000000 ) ) ;
#2110=LINE ( 'NONE', #640, #1184 ) ;
#2112=AXIS2_PLACEMENT_3D ( 'NONE', #10886, #2929, #12639 ) ;
#2129=CARTESIAN_POINT ( 'NONE',  ( -27.50000000000000711, 4.999999999999999112, 0.000000000000000000 ) ) ;
#2138=LINE ( 'NONE', #19928, #17039 ) ;
#2142=EDGE_LOOP ( 'NONE', ( #17794, #16886, #15579, #5598 ) ) ;
#2147=ORIENTED_EDGE ( 'NONE', *, *, #7241, .F. ) ;
#2149=LINE ( 'NONE', #8531, #12053 ) ;
#2162=LINE ( 'NONE', #2370, #7636 ) ;
#2164=CARTESIAN_POINT ( 'NONE',  ( 0.000000000000000000, 9.000000000000001776, 1.000000000000000000 ) ) ;
#2180=CARTESIAN_POINT ( 'NONE',  ( -5.999999999999999112, -7.500000000000047073, 9.999999999999998224 ) ) ;
#2192=AXIS2_PLACEMENT_3D ( 'NONE', #8146, #6982, #8958 ) ;
#2196=ORIENTED_EDGE ( 'NONE', *, *, #19330, .T. ) ;
#2199=LINE ( 'NONE', #6712, #16115 ) ;
#2201=ORIENTED_EDGE ( 'NONE', *, *, #2707, .T. ) ;
#2205=DIRECTION ( 'NONE',  ( 0.000000000000000000, 0.000000000000000000, 1.000000000000000000 ) ) ;
#2206=DIRECTION ( 'NONE',  ( -0.000000000000000000, -0.000000000000000000, -1.000000000000000000 ) ) ;
#2210=LINE ( 'NONE', #8592, #5043 ) ;
#2217=EDGE_CURVE ( 'NONE', #16327, #17198, #9616, .T. ) ;
#2220=ORIENTED_EDGE ( 'NONE', *, *, #13815, .T. ) ;
#2227=DIRECTION ( 'NONE',  ( 0.000000000000000000, -1.000000000000000000, 0.000000000000000000 ) ) ;
#2229=DIRECTION ( 'NONE',  ( 1.000000000000000000, 0.000000000000000000, -0.000000000000000000 ) ) ;
#2234=PLANE ( 'NONE',  #9369 ) ;
#2241=ADVANCED_FACE ( 'NONE', ( #18847 ), #6496, .T. ) ;
#2244=EDGE_CURVE ( 'NONE', #10986, #14610, #12547, .T. ) ;
#2248=VERTEX_POINT ( 'NONE', #19053 ) ;
#2254=EDGE_CURVE ( 'NONE', #8019, #14361, #4710, .T. ) ;
#2256=LINE ( 'NONE', #8448, #6316 ) ;
#2269=VECTOR ( 'NONE', #502, 1000.000000000000000 ) ;
#2271=CYLINDRICAL_SURFACE ( 'NONE', #15677, 0.4999999999999987232 ) ;
#2272=EDGE_LOOP ( 'NONE', ( #10405, #2024, #11415, #19506 ) ) ;
#2273=ORIENTED_EDGE ( 'NONE', *, *, #15162, .F. ) ;
#2277=ADVANCED_FACE ( 'NONE', ( #7005 ), #6698, .F. ) ;
#2279=VECTOR ( 'NONE', #4991, 1000.000000000000000 ) ;
#2281=DIRECTION ( 'NONE',  ( 0.000000000000000000, -0.000000000000000000, 1.000000000000000000 ) ) ;
#2283=DIRECTION ( 'NONE',  ( -1.000000000000000000, 0.000000000000000000, 0.000000000000000000 ) ) ;
#2294=CARTESIAN_POINT ( 'NONE',  ( 21.17243175760212637, 9.000000000000001776, 1.000000000000000000 ) ) ;
#2303=CARTESIAN_POINT ( 'NONE',  ( 24.50000000000000000, 0.000000000000000000, 1.000000000000000000 ) ) ;
#2306=LINE ( 'NONE', #5456, #3851 ) ;
#2313=LINE ( 'NONE', #8402, #9725 ) ;
#2318=EDGE_CURVE ( 'NONE', #1636, #2072, #14743, .T. ) ;
#2321=ORIENTED_EDGE ( 'NONE', *, *, #8111, .F. ) ;
#2327=VECTOR ( 'NONE', #18023, 1000.000000000000000 ) ;
#2328=ORIENTED_EDGE ( 'NONE', *, *, #7251, .F. ) ;
#2329=CARTESIAN_POINT ( 'NONE',  ( -20.92243175760212637, 9.000000000000001776, 0.000000000000000000 ) ) ;
#2333=EDGE_CURVE ( 'NONE', #2461, #7526, #5018, .T. ) ;
#2336=DIRECTION ( 'NONE',  ( 0.000000000000000000, -1.000000000000000000, 0.000000000000000000 ) ) ;
#2339=DIRECTION ( 'NONE',  ( 1.000000000000000000, 0.000000000000000000, 0.000000000000000000 ) ) ;
#2354=CARTESIAN_POINT ( 'NONE',  ( -25.29469207716615031, 0.000000000000000000, 0.000000000000000000 ) ) ;
#2356=CARTESIAN_POINT ( 'NONE',  ( -13.17791111847408025, 0.000000000000000000, 0.000000000000000000 ) ) ;
#2358=VECTOR ( 'NONE', #170, 1000.000000000000000 ) ;
#2364=ADVANCED_FACE ( 'NONE', ( #13069 ), #312, .F. ) ;
#2370=CARTESIAN_POINT ( 'NONE',  ( -19.48630159782011262, 0.000000000000000000, 0.000000000000000000 ) ) ;
#2379=VECTOR ( 'NONE', #18013, 1000.000000000000000 ) ;
#2381=FACE_OUTER_BOUND ( 'NONE', #2142, .T. ) ;
#2387=LINE ( 'NONE', #7419, #6618 ) ;
#2398=ORIENTED_EDGE ( 'NONE', *, *, #18015, .F. ) ;
#2406=EDGE_LOOP ( 'NONE', ( #4004, #9820, #889, #20540 ) ) ;
#2408=FACE_OUTER_BOUND ( 'NONE', #17328, .T. ) ;
#2410=AXIS2_PLACEMENT_3D ( 'NONE', #17620, #3290, #1521 ) ;
#2411=DIRECTION ( 'NONE',  ( -0.000000000000000000, -0.000000000000000000, -1.000000000000000000 ) ) ;
#2412=PLANE ( 'NONE',  #10370 ) ;
#2413=PLANE ( 'NONE',  #3971 ) ;
#2415=DIRECTION ( 'NONE',  ( 1.000000000000000000, 0.000000000000000000, 0.000000000000000000 ) ) ;
#2419=CARTESIAN_POINT ( 'NONE',  ( 0.000000000000000000, 4.999999999999999112, 1.000000000000000000 ) ) ;
#2423=DIRECTION ( 'NONE',  ( -1.000000000000000000, 0.000000000000000000, 0.000000000000000000 ) ) ;
#2432=EDGE_CURVE ( 'NONE', #14519, #13440, #3550, .T. ) ;
#2433=EDGE_LOOP ( 'NONE', ( #819, #7865, #10309, #10304 ) ) ;
#2441=CARTESIAN_POINT ( 'NONE',  ( -1.561130159782011306, 9.000000000000001776, 0.000000000000000000 ) ) ;
#2453=VERTEX_POINT ( 'NONE', #1780 ) ;
#2454=ORIENTED_EDGE ( 'NONE', *, *, #4226, .T. ) ;
#2459=ADVANCED_FACE ( 'NONE', ( #11598 ), #17983, .T. ) ;
#2461=VERTEX_POINT ( 'NONE', #8263 ) ;
#2462=PLANE ( 'NONE',  #5271 ) ;
#2478=FACE_OUTER_BOUND ( 'NONE', #13298, .T. ) ;
#2479=EDGE_CURVE ( 'NONE', #17198, #4223, #8882, .T. ) ;
#2485=DIRECTION ( 'NONE',  ( 1.000000000000000000, 0.000000000000000000, 0.000000000000000000 ) ) ;
#2487=DIRECTION ( 'NONE',  ( -0.000000000000000000, 0.000000000000000000, -1.000000000000000000 ) ) ;
#2488=CARTESIAN_POINT ( 'NONE',  ( 10.05565079891005631, 9.000000000000001776, 1.000000000000000000 ) ) ;
#2498=EDGE_CURVE ( 'NONE', #9688, #610, #8982, .T. ) ;
#2499=DIRECTION ( 'NONE',  ( 0.000000000000000000, 0.000000000000000000, 1.000000000000000000 ) ) ;
#2507=ORIENTED_EDGE ( 'NONE', *, *, #19909, .F. ) ;
#2508=CARTESIAN_POINT ( 'NONE',  ( -3.999999999999999112, -2.500000000000047518, 7.000000000000000000 ) ) ;
#2513=CARTESIAN_POINT ( 'NONE',  ( 25.54469207716615031, 9.000000000000001776, 0.000000000000000000 ) ) ;
#2518=CARTESIAN_POINT ( 'NONE',  ( 0.000000000000000000, 9.000000000000001776, 1.000000000000000000 ) ) ;
#2520=PLANE ( 'NONE',  #15720 ) ;
#2524=ORIENTED_EDGE ( 'NONE', *, *, #13066, .T. ) ;
#2528=ORIENTED_EDGE ( 'NONE', *, *, #3640, .F. ) ;
#2531=CARTESIAN_POINT ( 'NONE',  ( 0.000000000000000000, 4.999999999999999112, 1.000000000000000000 ) ) ;
#2540=CARTESIAN_POINT ( 'NONE',  ( 17.11324865405191176, -10.99999999999999645, 1.000000000000000000 ) ) ;
#2545=ORIENTED_EDGE ( 'NONE', *, *, #4304, .F. ) ;
#2546=VECTOR ( 'NONE', #1113, 1000.000000000000000 ) ;
#2551=ORIENTED_EDGE ( 'NONE', *, *, #13882, .F. ) ;
#2554=LINE ( 'NONE', #11866, #9386 ) ;
#2555=ORIENTED_EDGE ( 'NONE', *, *, #1486, .T. ) ;
#2556=ORIENTED_EDGE ( 'NONE', *, *, #1394, .T. ) ;
#2557=DIRECTION ( 'NONE',  ( 0.000000000000000000, 1.000000000000000000, -0.000000000000000000 ) ) ;
#2563=DIRECTION ( 'NONE',  ( 1.000000000000000000, 8.673617379884033500E-16, -0.000000000000000000 ) ) ;
#2564=CARTESIAN_POINT ( 'NONE',  ( 11.49178095869207006, 4.999999999999999112, 1.000000000000000000 ) ) ;
#2567=ADVANCED_FACE ( 'NONE', ( #7522 ), #18406, .T. ) ;
#2577=EDGE_CURVE ( 'NONE', #12897, #13753, #925, .T. ) ;
#2583=CARTESIAN_POINT ( 'NONE',  ( 25.54469207716615031, 9.000000000000001776, 1.000000000000000000 ) ) ;
#2589=CARTESIAN_POINT ( 'NONE',  ( 0.000000000000000000, 4.999999999999999112, 1.000000000000000000 ) ) ;
#2590=CARTESIAN_POINT ( 'NONE',  ( -1.561130159782011306, 4.999999999999999112, 0.000000000000000000 ) ) ;
#2593=FACE_OUTER_BOUND ( 'NONE', #3647, .T. ) ;
#2596=DIRECTION ( 'NONE',  ( -1.000000000000000000, 0.000000000000000000, 0.000000000000000000 ) ) ;
#2605=CARTESIAN_POINT ( 'NONE',  ( 4.247260319564023945, 0.000000000000000000, 0.000000000000000000 ) ) ;
#2607=VERTEX_POINT ( 'NONE', #15044 ) ;
#2624=VECTOR ( 'NONE', #19131, 1000.000000000000000 ) ;
#2628=EDGE_CURVE ( 'NONE', #9247, #9180, #10346, .T. ) ;
#2629=DIRECTION ( 'NONE',  ( -0.000000000000000000, 0.000000000000000000, -1.000000000000000000 ) ) ;
#2636=FACE_OUTER_BOUND ( 'NONE', #1256, .T. ) ;
#2643=VECTOR ( 'NONE', #7124, 1000.000000000000000 ) ;
#2647=CARTESIAN_POINT ( 'NONE',  ( 0.000000000000000000, 4.999999999999999112, 1.000000000000000000 ) ) ;
#2656=DIRECTION ( 'NONE',  ( 0.000000000000000000, -1.000000000000000000, 0.000000000000000000 ) ) ;
#2659=AXIS2_PLACEMENT_3D ( 'NONE', #4850, #3280, #11333 ) ;
#2660=ORIENTED_EDGE ( 'NONE', *, *, #3263, .F. ) ;
#2666=CARTESIAN_POINT ( 'NONE',  ( -5.433390479346035029, 4.999999999999999112, 0.000000000000000000 ) ) ;
#2667=AXIS2_PLACEMENT_3D ( 'NONE', #13167, #16514, #14841 ) ;
#2670=CARTESIAN_POINT ( 'NONE',  ( -14.00000000000000000, 0.000000000000000000, 0.5000000000000000000 ) ) ;
#2681=LINE ( 'NONE', #15538, #11625 ) ;
#2691=VECTOR ( 'NONE', #17232, 1000.000000000000000 ) ;
#2695=ORIENTED_EDGE ( 'NONE', *, *, #4274, .F. ) ;
#2697=VECTOR ( 'NONE', #19430, 1000.000000000000000 ) ;
#2698=AXIS2_PLACEMENT_3D ( 'NONE', #17310, #1010, #15745 ) ;
#2701=DIRECTION ( 'NONE',  ( 0.000000000000000000, -1.000000000000000000, 0.000000000000000000 ) ) ;
#2702=DIRECTION ( 'NONE',  ( -0.000000000000000000, -0.000000000000000000, -1.000000000000000000 ) ) ;
#2706=DIRECTION ( 'NONE',  ( 0.000000000000000000, 0.000000000000000000, -1.000000000000000000 ) ) ;
#2707=EDGE_CURVE ( 'NONE', #7093, #14252, #18711, .T. ) ;
#2712=VECTOR ( 'NONE', #20650, 1000.000000000000000 ) ;
#2713=VECTOR ( 'NONE', #14659, 1000.000000000000000 ) ;
#2721=ORIENTED_EDGE ( 'NONE', *, *, #9878, .T. ) ;
#2725=EDGE_CURVE ( 'NONE', #4209, #16676, #1831, .T. ) ;
#2727=ORIENTED_EDGE ( 'NONE', *, *, #6841, .F. ) ;
#2730=DIRECTION ( 'NONE',  ( -0.000000000000000000, -0.000000000000000000, -1.000000000000000000 ) ) ;
#2731=VECTOR ( 'NONE', #5285, 999.9999999999998863 ) ;
#2732=EDGE_CURVE ( 'NONE', #4209, #12230, #4862, .T. ) ;
#2733=PLANE ( 'NONE',  #11202 ) ;
#2735=EDGE_CURVE ( 'NONE', #14584, #15234, #17134, .T. ) ;
#2740=FACE_OUTER_BOUND ( 'NONE', #3282, .T. ) ;
#2745=ORIENTED_EDGE ( 'NONE', *, *, #2735, .T. ) ;
#2748=ORIENTED_EDGE ( 'NONE', *, *, #18015, .T. ) ;
#2749=EDGE_CURVE ( 'NONE', #4780, #5494, #20672, .T. ) ;
#2751=EDGE_CURVE ( 'NONE', #16350, #19789, #15942, .T. ) ;
#2770=ORIENTED_EDGE ( 'NONE', *, *, #13856, .F. ) ;
#2775=VECTOR ( 'NONE', #17585, 1000.000000000000000 ) ;
#2779=EDGE_CURVE ( 'NONE', #6813, #4981, #13015, .T. ) ;
#2781=CARTESIAN_POINT ( 'NONE',  ( -13.50000000000000178, -0.4999999999999987232, 1.000000000000000000 ) ) ;
#2783=VECTOR ( 'NONE', #12233, 1000.000000000000000 ) ;
#2784=CARTESIAN_POINT ( 'NONE',  ( 0.000000000000000000, 9.000000000000001776, 1.000000000000000000 ) ) ;
#2789=LINE ( 'NONE', #10345, #8749 ) ;
#2792=DIRECTION ( 'NONE',  ( 0.000000000000000000, 0.000000000000000000, -1.000000000000000000 ) ) ;
#2794=DIRECTION ( 'NONE',  ( 0.000000000000000000, 1.000000000000000000, -0.000000000000000000 ) ) ;
#2799=VERTEX_POINT ( 'NONE', #12907 ) ;
#2806=ORIENTED_EDGE ( 'NONE', *, *, #17901, .T. ) ;
#2811=DIRECTION ( 'NONE',  ( 0.000000000000000000, -1.000000000000000000, 0.000000000000000000 ) ) ;
#2812=DIRECTION ( 'NONE',  ( 0.000000000000000000, 1.000000000000000000, -0.000000000000000000 ) ) ;
#2818=EDGE_LOOP ( 'NONE', ( #12637, #1943, #2745, #8128 ) ) ;
#2822=ORIENTED_EDGE ( 'NONE', *, *, #14828, .T. ) ;
#2829=DIRECTION ( 'NONE',  ( 1.000000000000000000, 0.000000000000000000, -0.000000000000000000 ) ) ;
#2831=CYLINDRICAL_SURFACE ( 'NONE', #15797, 0.4999999999999987232 ) ;
#2834=CARTESIAN_POINT ( 'NONE',  ( -5.433390479346035029, 4.999999999999999112, 1.000000000000000000 ) ) ;
#2835=CARTESIAN_POINT ( 'NONE',  ( -20.00000000000000000, 0.000000000000000000, 1.000000000000000000 ) ) ;
#2840=ADVANCED_FACE ( 'NONE', ( #6644 ), #3197, .T. ) ;
#2843=AXIS2_PLACEMENT_3D ( 'NONE', #1164, #13907, #15688 ) ;
#2846=VERTEX_POINT ( 'NONE', #6446 ) ;
#2847=EDGE_CURVE ( 'NONE', #17347, #16469, #19311, .T. ) ;
#2852=ORIENTED_EDGE ( 'NONE', *, *, #9232, .F. ) ;
#2853=CARTESIAN_POINT ( 'NONE',  ( -18.98630159782011262, 9.000000000000001776, 0.000000000000000000 ) ) ;
#2855=CARTESIAN_POINT ( 'NONE',  ( -14.00000000000000000, 0.000000000000000000, 0.5000000000000000000 ) ) ;
#2858=CARTESIAN_POINT ( 'NONE',  ( 13.92791111847407848, 0.000000000000000000, 1.000000000000000000 ) ) ;
#2872=LINE ( 'NONE', #4746, #1040 ) ;
#2875=CARTESIAN_POINT ( 'NONE',  ( -11.74178095869206828, 4.999999999999999112, 0.000000000000000000 ) ) ;
#2881=CARTESIAN_POINT ( 'NONE',  ( 23.10856191738414012, 0.000000000000000000, 1.000000000000000000 ) ) ;
#2887=ADVANCED_FACE ( 'NONE', ( #5076 ), #11452, .F. ) ;
#2890=ADVANCED_FACE ( 'NONE', ( #5379 ), #2234, .F. ) ;
#2891=CARTESIAN_POINT ( 'NONE',  ( -1.561130159782011306, 0.000000000000000000, 0.000000000000000000 ) ) ;
#2905=EDGE_CURVE ( 'NONE', #16449, #11562, #2138, .T. ) ;
#2907=PLANE ( 'NONE',  #10323 ) ;
#2908=LINE ( 'NONE', #20696, #16000 ) ;
#2913=CIRCLE ( 'NONE', #13920, 2.999999999999999112 ) ;
#2915=SURFACE_STYLE_FILL_AREA ( #9399 ) ;
#2926=CARTESIAN_POINT ( 'NONE',  ( 0.000000000000000000, 9.000000000000001776, 1.000000000000000000 ) ) ;
#2927=EDGE_LOOP ( 'NONE', ( #15215, #19844, #18600, #10179 ) ) ;
#2929=DIRECTION ( 'NONE',  ( -0.9848077530122082424, -0.1736481776669295263, 0.000000000000000000 ) ) ;
#2933=CARTESIAN_POINT ( 'NONE',  ( -13.17791111847408025, 9.000000000000001776, 0.000000000000000000 ) ) ;
#2939=CARTESIAN_POINT ( 'NONE',  ( 9.830951894845298966, -2.500000000000047518, 7.000000000000000000 ) ) ;
#2944=VERTEX_POINT ( 'NONE', #8520 ) ;
#2947=ORIENTED_EDGE ( 'NONE', *, *, #4936, .T. ) ;
#2953=AXIS2_PLACEMENT_3D ( 'NONE', #9282, #3119, #14399 ) ;
#2959=CARTESIAN_POINT ( 'NONE',  ( 0.000000000000000000, 4.999999999999999112, 1.000000000000000000 ) ) ;
#2962=CARTESIAN_POINT ( 'NONE',  ( -5.433390479346035029, 9.000000000000001776, 0.000000000000000000 ) ) ;
#2975=CLOSED_SHELL ( 'NONE', ( #7499, #2277, #12051, #3012, #15989, #12541, #13547, #6853, #11164, #7868, #2890, #11870, #15055, #10182, #4383, #2567, #20489, #20113, #3888, #8779, #19760, #96, #8888, #13109, #6176, #12353, #5128, #20122, #13726, #18973, #6075, #4693, #7047, #10452, #2241, #6249, #12341, #5066, #15667, #16188, #17583, #19337, #5792, #3365, #20058, #2840, #15239, #6192, #3221, #20166, #16187, #13179, #11921, #2028, #18117, #4162, #3329, #19477, #14418, #9146, #13684, #9283, #17274, #11531, #15888, #15805, #9396, #20547, #1692, #17090, #4502, #12352, #15496, #15274, #8624, #15868, #10049, #14227, #19010, #20582, #10699, #9988, #10763, #9212, #18575, #14499, #758, #6487, #8773, #11011, #17860, #3679, #20006, #12084, #18058, #18480, #18817, #13181, #5716, #9299, #16222, #12729, #15373, #19384, #17874, #7187, #18926, #15924, #10371, #3115, #8774, #4527, #14986, #19902, #19712, #15773, #1450, #8140, #18315, #17029, #18698, #9732, #13808, #2459, #8251, #5820, #19453, #15121, #16508, #11804, #9007, #18742, #19854, #17348, #5578, #19942, #18438, #3515, #19866, #591, #18371, #2364, #14884, #10136, #2887, #12593, #12880, #6816 ) ) ;
#2977=VECTOR ( 'NONE', #14711, 1000.000000000000000 ) ;
#2978=ORIENTED_EDGE ( 'NONE', *, *, #12919, .F. ) ;
#2980=CIRCLE ( 'NONE', #20024, 0.4999999999999987232 ) ;
#2982=LINE ( 'NONE', #9869, #6091 ) ;
#2991=LINE ( 'NONE', #1423, #7183 ) ;
#2993=VECTOR ( 'NONE', #3390, 1000.000000000000000 ) ;
#2996=LINE ( 'NONE', #4560, #4660 ) ;
#3002=ORIENTED_EDGE ( 'NONE', *, *, #12679, .T. ) ;
#3012=ADVANCED_FACE ( 'NONE', ( #17695, #19489, #17900, #21, #16022 ), #2002, .F. ) ;
#3015=FACE_OUTER_BOUND ( 'NONE', #2433, .T. ) ;
#3018=DIRECTION ( 'NONE',  ( 0.000000000000000000, -0.000000000000000000, 1.000000000000000000 ) ) ;
#3029=VERTEX_POINT ( 'NONE', #17803 ) ;
#3033=ORIENTED_EDGE ( 'NONE', *, *, #12553, .T. ) ;
#3037=LINE ( 'NONE', #17463, #7464 ) ;
#3039=ORIENTED_EDGE ( 'NONE', *, *, #15226, .F. ) ;
#3043=VECTOR ( 'NONE', #9834, 1000.000000000000000 ) ;
#3044=FACE_OUTER_BOUND ( 'NONE', #11441, .T. ) ;
#3054=DIRECTION ( 'NONE',  ( -0.000000000000000000, -0.000000000000000000, -1.000000000000000000 ) ) ;
#3063=LINE ( 'NONE', #11211, #4769 ) ;
#3069=DIRECTION ( 'NONE',  ( 0.4999999999999950040, -0.8660254037844415942, 0.000000000000000000 ) ) ;
#3073=AXIS2_PLACEMENT_3D ( 'NONE', #20214, #7549, #12145 ) ;
#3085=DIRECTION ( 'NONE',  ( -1.000000000000000000, -0.000000000000000000, -0.000000000000000000 ) ) ;
#3086=ORIENTED_EDGE ( 'NONE', *, *, #1166, .T. ) ;
#3087=ORIENTED_EDGE ( 'NONE', *, *, #10578, .T. ) ;
#3092=CARTESIAN_POINT ( 'NONE',  ( 0.000000000000000000, 9.000000000000001776, 0.000000000000000000 ) ) ;
#3096=CARTESIAN_POINT ( 'NONE',  ( -27.50000000000000355, 3.000000000000000888, 1.000000000000000000 ) ) ;
#3099=CARTESIAN_POINT ( 'NONE',  ( 0.000000000000000000, 4.999999999999999112, 1.000000000000000000 ) ) ;
#3100=CARTESIAN_POINT ( 'NONE',  ( 0.000000000000000000, 0.000000000000000000, 1.000000000000000000 ) ) ;
#3107=ORIENTED_EDGE ( 'NONE', *, *, #16512, .F. ) ;
#3112=ORIENTED_EDGE ( 'NONE', *, *, #2479, .T. ) ;
#3115=ADVANCED_FACE ( 'NONE', ( #3367 ), #8388, .T. ) ;
#3119=DIRECTION ( 'NONE',  ( -1.000000000000000000, 0.000000000000000000, 0.000000000000000000 ) ) ;
#3125=LINE ( 'NONE', #11076, #13866 ) ;
#3128=ORIENTED_EDGE ( 'NONE', *, *, #7691, .T. ) ;
#3134=ORIENTED_EDGE ( 'NONE', *, *, #2318, .T. ) ;
#3135=DIRECTION ( 'NONE',  ( 0.000000000000000000, 1.000000000000000000, -0.000000000000000000 ) ) ;
#3137=ORIENTED_EDGE ( 'NONE', *, *, #6636, .T. ) ;
#3140=VERTEX_POINT ( 'NONE', #6610 ) ;
#3143=VECTOR ( 'NONE', #11902, 1000.000000000000000 ) ;
#3150=EDGE_CURVE ( 'NONE', #20018, #4438, #17587, .T. ) ;
#3154=CARTESIAN_POINT ( 'NONE',  ( 0.000000000000000000, 9.000000000000001776, 1.000000000000000000 ) ) ;
#3157=ORIENTED_EDGE ( 'NONE', *, *, #9533, .F. ) ;
#3159=CARTESIAN_POINT ( 'NONE',  ( -5.933390479346035029, 0.000000000000000000, 1.000000000000000000 ) ) ;
#3165=EDGE_CURVE ( 'NONE', #15422, #10048, #5700, .T. ) ;
#3182=PLANE ( 'NONE',  #4037 ) ;
#3184=ORIENTED_EDGE ( 'NONE', *, *, #1560, .T. ) ;
#3186=CARTESIAN_POINT ( 'NONE',  ( 0.000000000000000000, 9.000000000000001776, 1.000000000000000000 ) ) ;
#3189=FACE_OUTER_BOUND ( 'NONE', #16253, .T. ) ;
#3197=PLANE ( 'NONE',  #15035 ) ;
#3198=CARTESIAN_POINT ( 'NONE',  ( 27.50000000000000355, 3.000000000000000888, 1.000000000000000000 ) ) ;
#3209=VERTEX_POINT ( 'NONE', #16431 ) ;
#3210=ORIENTED_EDGE ( 'NONE', *, *, #927, .T. ) ;
#3212=EDGE_LOOP ( 'NONE', ( #10514, #13137, #15398, #3641 ) ) ;
#3213=DIRECTION ( 'NONE',  ( 0.000000000000000000, 0.000000000000000000, 1.000000000000000000 ) ) ;
#3214=ORIENTED_EDGE ( 'NONE', *, *, #871, .F. ) ;
#3215=DIRECTION ( 'NONE',  ( -1.000000000000000000, 0.000000000000000000, 0.000000000000000000 ) ) ;
#3216=EDGE_CURVE ( 'NONE', #9688, #2075, #15171, .T. ) ;
#3221=ADVANCED_FACE ( 'NONE', ( #7229 ), #11924, .T. ) ;
#3222=EDGE_CURVE ( 'NONE', #12251, #18418, #3673, .T. ) ;
#3227=LINE ( 'NONE', #3326, #16429 ) ;
#3232=ORIENTED_EDGE ( 'NONE', *, *, #15898, .T. ) ;
#3233=LINE ( 'NONE', #11086, #11275 ) ;
#3234=ORIENTED_EDGE ( 'NONE', *, *, #18519, .T. ) ;
#3240=CARTESIAN_POINT ( 'NONE',  ( -7.369520639128046113, 9.000000000000001776, 0.000000000000000000 ) ) ;
#3246=DIRECTION ( 'NONE',  ( 1.000000000000000000, 0.000000000000000000, 0.000000000000000000 ) ) ;
#3255=AXIS2_PLACEMENT_3D ( 'NONE', #7664, #969, #1391 ) ;
#3257=ORIENTED_EDGE ( 'NONE', *, *, #7457, .F. ) ;
#3259=CARTESIAN_POINT ( 'NONE',  ( -3.997260319564023501, 4.999999999999999112, 0.000000000000000000 ) ) ;
#3263=EDGE_CURVE ( 'NONE', #6051, #42, #16842, .T. ) ;
#3265=DIRECTION ( 'NONE',  ( 0.000000000000000000, 1.000000000000000000, 0.000000000000000000 ) ) ;
#3268=CARTESIAN_POINT ( 'NONE',  ( -22.85856191738413656, 9.000000000000001776, 1.000000000000000000 ) ) ;
#3269=PLANE ( 'NONE',  #17416 ) ;
#3277=ORIENTED_EDGE ( 'NONE', *, *, #12484, .T. ) ;
#3280=DIRECTION ( 'NONE',  ( 1.000000000000000000, 0.000000000000000000, -0.000000000000000000 ) ) ;
#3282=EDGE_LOOP ( 'NONE', ( #4373, #558, #13437, #1279 ) ) ;
#3289=DIRECTION ( 'NONE',  ( 1.000000000000000000, 0.000000000000000000, -0.000000000000000000 ) ) ;
#3290=DIRECTION ( 'NONE',  ( 0.000000000000000000, 1.000000000000000000, 0.000000000000000000 ) ) ;
#3291=DIRECTION ( 'NONE',  ( 0.000000000000000000, 5.204170427930421283E-15, 1.000000000000000000 ) ) ;
#3302=VECTOR ( 'NONE', #8218, 1000.000000000000000 ) ;
#3305=CARTESIAN_POINT ( 'NONE',  ( 25.04469207716615031, 9.000000000000001776, 1.000000000000000000 ) ) ;
#3316=VECTOR ( 'NONE', #16099, 1000.000000000000000 ) ;
#3320=DIRECTION ( 'NONE',  ( 1.000000000000000000, 0.000000000000000000, 0.000000000000000000 ) ) ;
#3322=PLANE ( 'NONE',  #2192 ) ;
#3326=CARTESIAN_POINT ( 'NONE',  ( 7.619520639128047002, 0.000000000000000000, 1.000000000000000000 ) ) ;
#3328=ORIENTED_EDGE ( 'NONE', *, *, #13242, .F. ) ;
#3329=ADVANCED_FACE ( 'NONE', ( #5345 ), #2412, .T. ) ;
#3338=DIRECTION ( 'NONE',  ( 1.000000000000000000, 0.000000000000000000, 0.000000000000000000 ) ) ;
#3339=EDGE_CURVE ( 'NONE', #15255, #4739, #8901, .T. ) ;
#3340=EDGE_CURVE ( 'NONE', #8718, #13902, #12029, .T. ) ;
#3345=CARTESIAN_POINT ( 'NONE',  ( 26.79469207716614676, 9.000000000000001776, 0.000000000000000000 ) ) ;
#3353=CARTESIAN_POINT ( 'NONE',  ( 0.000000000000000000, 9.000000000000001776, 1.000000000000000000 ) ) ;
#3358=ORIENTED_EDGE ( 'NONE', *, *, #6057, .F. ) ;
#3365=ADVANCED_FACE ( 'NONE', ( #20103 ), #5766, .T. ) ;
#3366=EDGE_CURVE ( 'NONE', #9600, #2799, #8587, .T. ) ;
#3367=FACE_OUTER_BOUND ( 'NONE', #331, .T. ) ;
#3372=PLANE ( 'NONE',  #18036 ) ;
#3376=CARTESIAN_POINT ( 'NONE',  ( 21.67243175760212637, 4.999999999999999112, 1.000000000000000000 ) ) ;
#3382=VECTOR ( 'NONE', #16870, 1000.000000000000000 ) ;
#3383=EDGE_CURVE ( 'NONE', #2461, #20415, #7025, .T. ) ;
#3390=DIRECTION ( 'NONE',  ( 8.673617379884033500E-16, -1.000000000000000000, 0.000000000000000000 ) ) ;
#3391=EDGE_LOOP ( 'NONE', ( #15808, #5113, #10155, #11308 ) ) ;
#3393=LINE ( 'NONE', #3186, #7762 ) ;
#3409=ORIENTED_EDGE ( 'NONE', *, *, #6382, .F. ) ;
#3413=ORIENTED_EDGE ( 'NONE', *, *, #6925, .T. ) ;
#3415=VECTOR ( 'NONE', #6864, 1000.000000000000000 ) ;
#3417=VERTEX_POINT ( 'NONE', #15637 ) ;
#3418=DIRECTION ( 'NONE',  ( 0.000000000000000000, 1.000000000000000000, 0.000000000000000000 ) ) ;
#3419=VECTOR ( 'NONE', #4939, 1000.000000000000000 ) ;
#3428=VECTOR ( 'NONE', #20442, 1000.000000000000000 ) ;
#3431=DIRECTION ( 'NONE',  ( 1.000000000000000000, 0.000000000000000000, -0.000000000000000000 ) ) ;
#3442=VECTOR ( 'NONE', #3468, 1000.000000000000000 ) ;
#3444=VERTEX_POINT ( 'NONE', #13863 ) ;
#3464=CARTESIAN_POINT ( 'NONE',  ( 15.36404127825609400, 4.999999999999999112, 0.000000000000000000 ) ) ;
#3467=ORIENTED_EDGE ( 'NONE', *, *, #8721, .F. ) ;
#3468=DIRECTION ( 'NONE',  ( 0.000000000000000000, 1.000000000000000000, -0.000000000000000000 ) ) ;
#3469=CARTESIAN_POINT ( 'NONE',  ( -24.50000000000000000, 3.000000000000000888, 0.000000000000000000 ) ) ;
#3473=LINE ( 'NONE', #17905, #14731 ) ;
#3477=DIRECTION ( 'NONE',  ( 1.000000000000000000, 0.000000000000000000, 0.000000000000000000 ) ) ;
#3484=LINE ( 'NONE', #9762, #12382 ) ;
#3500=CARTESIAN_POINT ( 'NONE',  ( 3.747260319564023501, 9.000000000000001776, 0.000000000000000000 ) ) ;
#3502=CARTESIAN_POINT ( 'NONE',  ( 0.000000000000000000, 4.999999999999999112, 1.000000000000000000 ) ) ;
#3503=CARTESIAN_POINT ( 'NONE',  ( 13.00000000000000355, 7.806255641895631925E-15, 1.000000000000000000 ) ) ;
#3512=DIRECTION ( 'NONE',  ( 1.000000000000000000, 0.000000000000000000, 0.000000000000000000 ) ) ;
#3514=CIRCLE ( 'NONE', #20607, 0.4999999999999987232 ) ;
#3515=ADVANCED_FACE ( 'NONE', ( #13762 ), #9371, .T. ) ;
#3519=ORIENTED_EDGE ( 'NONE', *, *, #14510, .T. ) ;
#3521=EDGE_LOOP ( 'NONE', ( #18263, #4190, #8551, #9985 ) ) ;
#3524=EDGE_CURVE ( 'NONE', #9059, #4330, #17005, .T. ) ;
#3534=ORIENTED_EDGE ( 'NONE', *, *, #17568, .F. ) ;
#3540=CARTESIAN_POINT ( 'NONE',  ( 2.311130159782011972, 9.000000000000001776, 1.000000000000000000 ) ) ;
#3550=LINE ( 'NONE', #618, #5335 ) ;
#3557=EDGE_CURVE ( 'NONE', #5157, #2020, #9068, .T. ) ;
#3560=ORIENTED_EDGE ( 'NONE', *, *, #6746, .T. ) ;
#3563=FACE_OUTER_BOUND ( 'NONE', #9994, .T. ) ;
#3565=ORIENTED_EDGE ( 'NONE', *, *, #9382, .F. ) ;
#3568=DIRECTION ( 'NONE',  ( -0.000000000000000000, 0.000000000000000000, -1.000000000000000000 ) ) ;
#3571=DIRECTION ( 'NONE',  ( -0.000000000000000000, -0.000000000000000000, -1.000000000000000000 ) ) ;
#3572=CARTESIAN_POINT ( 'NONE',  ( 19.23630159782011617, 9.000000000000001776, 0.000000000000000000 ) ) ;
#3577=LINE ( 'NONE', #3793, #6356 ) ;
#3579=CARTESIAN_POINT ( 'NONE',  ( 0.000000000000000000, 9.000000000000001776, 1.000000000000000000 ) ) ;
#3582=ORIENTED_EDGE ( 'NONE', *, *, #15346, .F. ) ;
#3589=ORIENTED_EDGE ( 'NONE', *, *, #553, .F. ) ;
#3592=VECTOR ( 'NONE', #2702, 1000.000000000000000 ) ;
#3593=EDGE_CURVE ( 'NONE', #19731, #19600, #15440, .T. ) ;
#3595=CARTESIAN_POINT ( 'NONE',  ( -25.29469207716615031, 4.999999999999999112, 0.000000000000000000 ) ) ;
#3598=DIRECTION ( 'NONE',  ( 0.000000000000000000, -0.000000000000000000, 1.000000000000000000 ) ) ;
#3601=FACE_OUTER_BOUND ( 'NONE', #997, .T. ) ;
#3608=ORIENTED_EDGE ( 'NONE', *, *, #16361, .F. ) ;
#3612=VERTEX_POINT ( 'NONE', #13963 ) ;
#3616=ORIENTED_EDGE ( 'NONE', *, *, #7346, .F. ) ;
#3617=LINE ( 'NONE', #18057, #16443 ) ;
#3623=CARTESIAN_POINT ( 'NONE',  ( -18.98630159782011262, 4.999999999999999112, 0.000000000000000000 ) ) ;
#3625=AXIS2_PLACEMENT_3D ( 'NONE', #12521, #3215, #4676 ) ;
#3626=EDGE_CURVE ( 'NONE', #14595, #14589, #17623, .T. ) ;
#3627=AXIS2_PLACEMENT_3D ( 'NONE', #20137, #20336, #10710 ) ;
#3630=DIRECTION ( 'NONE',  ( 0.000000000000000000, -1.000000000000000000, 0.000000000000000000 ) ) ;
#3638=EDGE_CURVE ( 'NONE', #6239, #8745, #14485, .T. ) ;
#3639=DIRECTION ( 'NONE',  ( 0.000000000000000000, -1.000000000000000000, 0.000000000000000000 ) ) ;
#3640=EDGE_CURVE ( 'NONE', #18418, #19600, #6646, .T. ) ;
#3641=ORIENTED_EDGE ( 'NONE', *, *, #4872, .T. ) ;
#3647=EDGE_LOOP ( 'NONE', ( #8554, #1181, #6661, #10410, #15244, #274, #11069, #4006, #580, #16277 ) ) ;
#3654=VECTOR ( 'NONE', #16460, 1000.000000000000000 ) ;
#3659=CARTESIAN_POINT ( 'NONE',  ( 0.000000000000000000, 9.000000000000001776, 0.000000000000000000 ) ) ;
#3660=CARTESIAN_POINT ( 'NONE',  ( 26.04469207716615031, 9.000000000000001776, 1.000000000000000000 ) ) ;
#3664=ORIENTED_EDGE ( 'NONE', *, *, #3786, .F. ) ;
#3665=EDGE_CURVE ( 'NONE', #13753, #10392, #12812, .T. ) ;
#3669=CARTESIAN_POINT ( 'NONE',  ( -11.74178095869206828, 4.999999999999999112, 1.000000000000000000 ) ) ;
#3671=LINE ( 'NONE', #746, #2096 ) ;
#3673=LINE ( 'NONE', #11824, #11367 ) ;
#3679=ADVANCED_FACE ( 'NONE', ( #8315 ), #20674, .T. ) ;
#3688=VECTOR ( 'NONE', #16770, 1000.000000000000000 ) ;
#3694=VECTOR ( 'NONE', #12043, 1000.000000000000000 ) ;
#3696=AXIS2_PLACEMENT_3D ( 'NONE', #20370, #20480, #18692 ) ;
#3699=DIRECTION ( 'NONE',  ( -0.000000000000000000, -0.000000000000000000, -1.000000000000000000 ) ) ;
#3702=CARTESIAN_POINT ( 'NONE',  ( -24.50000000000000000, 3.000000000000000888, 1.000000000000000000 ) ) ;
#3705=FACE_OUTER_BOUND ( 'NONE', #10422, .T. ) ;
#3707=DIRECTION ( 'NONE',  ( 1.000000000000000000, 0.000000000000000000, 0.000000000000000000 ) ) ;
#3709=EDGE_CURVE ( 'NONE', #20470, #17483, #12709, .T. ) ;
#3710=DIRECTION ( 'NONE',  ( 0.000000000000000000, -1.000000000000000000, 0.000000000000000000 ) ) ;
#3714=AXIS2_PLACEMENT_3D ( 'NONE', #9689, #5187, #6660 ) ;
#3716=VERTEX_POINT ( 'NONE', #3503 ) ;
#3720=VERTEX_POINT ( 'NONE', #12600 ) ;
#3723=ORIENTED_EDGE ( 'NONE', *, *, #4954, .F. ) ;
#3724=LINE ( 'NONE', #484, #13722 ) ;
#3726=DIRECTION ( 'NONE',  ( 1.000000000000000000, 0.000000000000000000, 0.000000000000000000 ) ) ;
#3731=DIRECTION ( 'NONE',  ( -0.000000000000000000, -0.000000000000000000, -1.000000000000000000 ) ) ;
#3747=EDGE_CURVE ( 'NONE', #1300, #8663, #4225, .T. ) ;
#3749=DIRECTION ( 'NONE',  ( -1.000000000000000000, 0.000000000000000000, 0.000000000000000000 ) ) ;
#3752=VERTEX_POINT ( 'NONE', #9345 ) ;
#3755=CARTESIAN_POINT ( 'NONE',  ( 23.60856191738414012, 9.000000000000001776, 1.000000000000000000 ) ) ;
#3756=VECTOR ( 'NONE', #6331, 1000.000000000000000 ) ;
#3761=EDGE_CURVE ( 'NONE', #12230, #5259, #10507, .T. ) ;
#3763=CARTESIAN_POINT ( 'NONE',  ( -23.35856191738413656, 0.000000000000000000, 1.000000000000000000 ) ) ;
#3772=VERTEX_POINT ( 'NONE', #7375 ) ;
#3780=CARTESIAN_POINT ( 'NONE',  ( 11.49178095869207006, 0.000000000000000000, 1.000000000000000000 ) ) ;
#3781=FACE_OUTER_BOUND ( 'NONE', #11056, .T. ) ;
#3783=CARTESIAN_POINT ( 'NONE',  ( -3.997260319564023501, 0.000000000000000000, 1.000000000000000000 ) ) ;
#3786=EDGE_CURVE ( 'NONE', #999, #7456, #15722, .T. ) ;
#3791=CARTESIAN_POINT ( 'NONE',  ( -9.805650798910056309, 0.000000000000000000, 1.000000000000000000 ) ) ;
#3793=CARTESIAN_POINT ( 'NONE',  ( -15.61404127825609223, 0.000000000000000000, 0.000000000000000000 ) ) ;
#3801=ORIENTED_EDGE ( 'NONE', *, *, #1988, .T. ) ;
#3804=DIRECTION ( 'NONE',  ( 0.7071067811865475727, 0.000000000000000000, -0.7071067811865475727 ) ) ;
#3810=LINE ( 'NONE', #16261, #4708 ) ;
#3812=DIRECTION ( 'NONE',  ( 0.000000000000000000, -0.000000000000000000, 1.000000000000000000 ) ) ;
#3822=ORIENTED_EDGE ( 'NONE', *, *, #4238, .F. ) ;
#3823=VERTEX_POINT ( 'NONE', #12483 ) ;
#3829=ORIENTED_EDGE ( 'NONE', *, *, #2577, .F. ) ;
#3830=DIRECTION ( 'NONE',  ( 0.000000000000000000, -0.000000000000000000, 1.000000000000000000 ) ) ;
#3844=DIRECTION ( 'NONE',  ( 0.000000000000000000, 0.000000000000000000, 1.000000000000000000 ) ) ;
#3845=DIRECTION ( 'NONE',  ( -0.4999999999999947820, -0.8660254037844415942, 0.000000000000000000 ) ) ;
#3846=VECTOR ( 'NONE', #20364, 1000.000000000000000 ) ;
#3851=VECTOR ( 'NONE', #538, 1000.000000000000000 ) ;
#3852=ORIENTED_EDGE ( 'NONE', *, *, #12470, .T. ) ;
#3853=LINE ( 'NONE', #3952, #11642 ) ;
#3860=FACE_OUTER_BOUND ( 'NONE', #18577, .T. ) ;
#3865=VERTEX_POINT ( 'NONE', #10922 ) ;
#3871=EDGE_LOOP ( 'NONE', ( #2528, #78, #7484, #15377 ) ) ;
#3876=EDGE_CURVE ( 'NONE', #9549, #10573, #20341, .T. ) ;
#3877=DIRECTION ( 'NONE',  ( 0.000000000000000000, 1.000000000000000000, -0.000000000000000000 ) ) ;
#3878=CARTESIAN_POINT ( 'NONE',  ( -5.433390479346035029, 9.000000000000001776, 1.000000000000000000 ) ) ;
#3879=DIRECTION ( 'NONE',  ( 1.000000000000000000, 0.000000000000000000, 0.000000000000000000 ) ) ;
#3881=DIRECTION ( 'NONE',  ( 1.000000000000000000, 0.000000000000000000, -0.000000000000000000 ) ) ;
#3888=ADVANCED_FACE ( 'NONE', ( #9044 ), #15415, .T. ) ;
#3897=VECTOR ( 'NONE', #11948, 1000.000000000000000 ) ;
#3898=CARTESIAN_POINT ( 'NONE',  ( 0.000000000000000000, 4.999999999999999112, 1.000000000000000000 ) ) ;
#3899=ORIENTED_EDGE ( 'NONE', *, *, #10755, .F. ) ;
#3901=ORIENTED_EDGE ( 'NONE', *, *, #11498, .F. ) ;
#3902=EDGE_CURVE ( 'NONE', #14893, #4330, #20456, .T. ) ;
#3903=LINE ( 'NONE', #16552, #5443 ) ;
#3921=PLANE ( 'NONE',  #5714 ) ;
#3924=LINE ( 'NONE', #2354, #19802 ) ;
#3925=ORIENTED_EDGE ( 'NONE', *, *, #5034, .F. ) ;
#3929=LINE ( 'NONE', #20053, #6664 ) ;
#3930=DIRECTION ( 'NONE',  ( 1.000000000000000000, 0.000000000000000000, 0.000000000000000000 ) ) ;
#3935=LINE ( 'NONE', #493, #20664 ) ;
#3944=VERTEX_POINT ( 'NONE', #19293 ) ;
#3945=VECTOR ( 'NONE', #4277, 1000.000000000000000 ) ;
#3946=LINE ( 'NONE', #19962, #8281 ) ;
#3952=CARTESIAN_POINT ( 'NONE',  ( -21.42243175760212637, 0.000000000000000000, 1.000000000000000000 ) ) ;
#3956=LINE ( 'NONE', #10965, #16041 ) ;
#3968=AXIS2_PLACEMENT_3D ( 'NONE', #14284, #6359, #18064 ) ;
#3971=AXIS2_PLACEMENT_3D ( 'NONE', #16432, #19797, #11925 ) ;
#3980=CARTESIAN_POINT ( 'NONE',  ( 13.50000000000000178, 7.806255641895631925E-15, 2.000000000000000000 ) ) ;
#3981=CARTESIAN_POINT ( 'NONE',  ( 0.000000000000000000, 4.999999999999999112, 1.000000000000000000 ) ) ;
#3982=DIRECTION ( 'NONE',  ( 0.000000000000000000, -1.000000000000000000, 0.000000000000000000 ) ) ;
#3985=DIRECTION ( 'NONE',  ( 1.000000000000000000, 0.000000000000000000, 0.000000000000000000 ) ) ;
#3987=VECTOR ( 'NONE', #14617, 1000.000000000000000 ) ;
#3993=EDGE_CURVE ( 'NONE', #14460, #12662, #3484, .T. ) ;
#3998=ORIENTED_EDGE ( 'NONE', *, *, #6286, .T. ) ;
#4004=ORIENTED_EDGE ( 'NONE', *, *, #10270, .F. ) ;
#4006=ORIENTED_EDGE ( 'NONE', *, *, #13739, .F. ) ;
#4017=FACE_OUTER_BOUND ( 'NONE', #20255, .T. ) ;
#4020=ORIENTED_EDGE ( 'NONE', *, *, #8876, .F. ) ;
#4029=ORIENTED_EDGE ( 'NONE', *, *, #18173, .T. ) ;
#4030=ORIENTED_EDGE ( 'NONE', *, *, #6057, .T. ) ;
#4031=PLANE ( 'NONE',  #17417 ) ;
#4034=EDGE_CURVE ( 'NONE', #4780, #1844, #14563, .T. ) ;
#4035=VECTOR ( 'NONE', #17061, 1000.000000000000000 ) ;
#4036=ORIENTED_EDGE ( 'NONE', *, *, #7162, .F. ) ;
#4037=AXIS2_PLACEMENT_3D ( 'NONE', #4447, #4543, #7684 ) ;
#4038=FACE_OUTER_BOUND ( 'NONE', #12818, .T. ) ;
#4048=EDGE_CURVE ( 'NONE', #14054, #20705, #8197, .T. ) ;
#4058=CARTESIAN_POINT ( 'NONE',  ( -15.11404127825609223, 0.000000000000000000, 1.000000000000000000 ) ) ;
#4059=DIRECTION ( 'NONE',  ( -0.000000000000000000, -0.000000000000000000, -1.000000000000000000 ) ) ;
#4064=CARTESIAN_POINT ( 'NONE',  ( -4.999999999999998224, -2.500000000000047518, 9.999999999999998224 ) ) ;
#4065=CARTESIAN_POINT ( 'NONE',  ( 13.00000000000000355, 7.806255641895631925E-15, 2.000000000000000000 ) ) ;
#4067=LINE ( 'NONE', #4267, #12028 ) ;
#4069=VECTOR ( 'NONE', #13961, 1000.000000000000000 ) ;
#4076=CARTESIAN_POINT ( 'NONE',  ( 0.000000000000000000, 4.999999999999999112, 1.000000000000000000 ) ) ;
#4079=LINE ( 'NONE', #5648, #971 ) ;
#4080=ORIENTED_EDGE ( 'NONE', *, *, #12578, .T. ) ;
#4083=CARTESIAN_POINT ( 'NONE',  ( 3.999999999999999112, -7.500000000000047073, 7.000000000000000000 ) ) ;
#4086=AXIS2_PLACEMENT_3D ( 'NONE', #7917, #3418, #6662 ) ;
#4090=LINE ( 'NONE', #15065, #20007 ) ;
#4095=DIRECTION ( 'NONE',  ( -0.000000000000000000, -0.000000000000000000, -1.000000000000000000 ) ) ;
#4110=DIRECTION ( 'NONE',  ( 0.000000000000000000, -1.000000000000000000, 0.000000000000000000 ) ) ;
#4111=VECTOR ( 'NONE', #8387, 1000.000000000000000 ) ;
#4116=LINE ( 'NONE', #12474, #17071 ) ;
#4132=ORIENTED_EDGE ( 'NONE', *, *, #12158, .F. ) ;
#4138=ORIENTED_EDGE ( 'NONE', *, *, #6597, .F. ) ;
#4139=LINE ( 'NONE', #15320, #18012 ) ;
#4146=CARTESIAN_POINT ( 'NONE',  ( -13.67791111847408025, 4.999999999999999112, 1.000000000000000000 ) ) ;
#4148=LINE ( 'NONE', #10742, #12705 ) ;
#4162=ADVANCED_FACE ( 'NONE', ( #12889 ), #8294, .T. ) ;
#4164=ORIENTED_EDGE ( 'NONE', *, *, #17052, .F. ) ;
#4167=EDGE_CURVE ( 'NONE', #9694, #16571, #8406, .T. ) ;
#4169=DIRECTION ( 'NONE',  ( 0.000000000000000000, 1.000000000000000000, 0.000000000000000000 ) ) ;
#4170=DIRECTION ( 'NONE',  ( -1.000000000000000000, 0.000000000000000000, -0.000000000000000000 ) ) ;
#4171=CARTESIAN_POINT ( 'NONE',  ( 25.04469207716615031, 0.000000000000000000, 1.000000000000000000 ) ) ;
#4187=EDGE_LOOP ( 'NONE', ( #15880, #14734, #14736, #13079 ) ) ;
#4190=ORIENTED_EDGE ( 'NONE', *, *, #6734, .F. ) ;
#4200=EDGE_CURVE ( 'NONE', #19645, #10336, #7057, .T. ) ;
#4209=VERTEX_POINT ( 'NONE', #1928 ) ;
#4210=LINE ( 'NONE', #15400, #8450 ) ;
#4212=VECTOR ( 'NONE', #13653, 1000.000000000000000 ) ;
#4219=DIRECTION ( 'NONE',  ( 0.000000000000000000, 0.000000000000000000, 1.000000000000000000 ) ) ;
#4223=VERTEX_POINT ( 'NONE', #3500 ) ;
#4225=LINE ( 'NONE', #17286, #4372 ) ;
#4226=EDGE_CURVE ( 'NONE', #18281, #11254, #776, .T. ) ;
#4238=EDGE_CURVE ( 'NONE', #9082, #12662, #14990, .T. ) ;
#4239=DIRECTION ( 'NONE',  ( 0.000000000000000000, 0.000000000000000000, 1.000000000000000000 ) ) ;
#4247=DIRECTION ( 'NONE',  ( 1.000000000000000000, 0.000000000000000000, 0.000000000000000000 ) ) ;
#4251=LINE ( 'NONE', #15133, #4212 ) ;
#4258=ORIENTED_EDGE ( 'NONE', *, *, #821, .T. ) ;
#4264=DIRECTION ( 'NONE',  ( 0.000000000000000000, 1.000000000000000000, 0.000000000000000000 ) ) ;
#4265=CARTESIAN_POINT ( 'NONE',  ( 3.747260319564023501, 0.000000000000000000, 1.000000000000000000 ) ) ;
#4267=CARTESIAN_POINT ( 'NONE',  ( 1.811130159782011528, 4.999999999999999112, 1.000000000000000000 ) ) ;
#4269=CARTESIAN_POINT ( 'NONE',  ( -20.00000000000000000, -6.000000000000000000, 2.000000000000000000 ) ) ;
#4272=VECTOR ( 'NONE', #16203, 1000.000000000000000 ) ;
#4274=EDGE_CURVE ( 'NONE', #6051, #19095, #18037, .T. ) ;
#4275=EDGE_LOOP ( 'NONE', ( #7845, #2978, #8345, #16987 ) ) ;
#4276=EDGE_CURVE ( 'NONE', #20415, #7096, #3810, .T. ) ;
#4277=DIRECTION ( 'NONE',  ( -0.000000000000000000, -0.000000000000000000, -1.000000000000000000 ) ) ;
#4278=LINE ( 'NONE', #15468, #9418 ) ;
#4286=PRESENTATION_STYLE_ASSIGNMENT (( #12442 ) ) ;
#4287=ORIENTED_EDGE ( 'NONE', *, *, #7398, .F. ) ;
#4295=CARTESIAN_POINT ( 'NONE',  ( 0.000000000000000000, 4.999999999999999112, 1.000000000000000000 ) ) ;
#4302=EDGE_CURVE ( 'NONE', #4697, #7456, #5269, .T. ) ;
#4303=VECTOR ( 'NONE', #1931, 1000.000000000000000 ) ;
#4304=EDGE_CURVE ( 'NONE', #5740, #15982, #14687, .T. ) ;
#4309=ORIENTED_EDGE ( 'NONE', *, *, #16551, .T. ) ;
#4316=VECTOR ( 'NONE', #7495, 1000.000000000000000 ) ;
#4319=VECTOR ( 'NONE', #11914, 1000.000000000000000 ) ;
#4320=AXIS2_PLACEMENT_3D ( 'NONE', #10523, #10620, #8947 ) ;
#4323=CARTESIAN_POINT ( 'NONE',  ( 0.000000000000000000, 4.999999999999999112, 1.000000000000000000 ) ) ;
#4324=DIRECTION ( 'NONE',  ( 0.000000000000000000, 1.000000000000000000, 0.000000000000000000 ) ) ;
#4325=LINE ( 'NONE', #17081, #3688 ) ;
#4327=DIRECTION ( 'NONE',  ( 0.000000000000000000, -1.000000000000000000, 0.000000000000000000 ) ) ;
#4330=VERTEX_POINT ( 'NONE', #366 ) ;
#4333=CARTESIAN_POINT ( 'NONE',  ( 26.04469207716615031, 4.999999999999999112, 1.000000000000000000 ) ) ;
#4341=ORIENTED_EDGE ( 'NONE', *, *, #7234, .T. ) ;
#4349=CARTESIAN_POINT ( 'NONE',  ( -20.00000000000000000, -6.000000000000000000, 2.000000000000000000 ) ) ;
#4350=EDGE_CURVE ( 'NONE', #20018, #5573, #19613, .T. ) ;
#4358=DIRECTION ( 'NONE',  ( 1.000000000000000000, 0.000000000000000000, 0.000000000000000000 ) ) ;
#4368=DIRECTION ( 'NONE',  ( 1.000000000000000000, -0.000000000000000000, -0.000000000000000000 ) ) ;
#4371=VECTOR ( 'NONE', #684, 1000.000000000000000 ) ;
#4372=VECTOR ( 'NONE', #18464, 1000.000000000000000 ) ;
#4373=ORIENTED_EDGE ( 'NONE', *, *, #4048, .F. ) ;
#4375=DIRECTION ( 'NONE',  ( 0.8660254037844415942, 0.4999999999999950040, -0.000000000000000000 ) ) ;
#4379=CARTESIAN_POINT ( 'NONE',  ( -25.29469207716615031, 0.000000000000000000, 1.000000000000000000 ) ) ;
#4380=CARTESIAN_POINT ( 'NONE',  ( 7.619520639128047002, 9.000000000000001776, 1.000000000000000000 ) ) ;
#4382=EDGE_CURVE ( 'NONE', #14130, #14133, #19518, .T. ) ;
#4383=ADVANCED_FACE ( 'NONE', ( #5169 ), #14792, .T. ) ;
#4388=VECTOR ( 'NONE', #9336, 1000.000000000000000 ) ;
#4398=LINE ( 'NONE', #6073, #6584 ) ;
#4401=ORIENTED_EDGE ( 'NONE', *, *, #17788, .T. ) ;
#4404=CARTESIAN_POINT ( 'NONE',  ( 23.10856191738414012, 0.000000000000000000, 1.000000000000000000 ) ) ;
#4414=EDGE_CURVE ( 'NONE', #9600, #17347, #10188, .T. ) ;
#4415=AXIS2_PLACEMENT_3D ( 'NONE', #6463, #1537, #11362 ) ;
#4433=DIRECTION ( 'NONE',  ( -0.000000000000000000, -0.000000000000000000, -1.000000000000000000 ) ) ;
#4434=CARTESIAN_POINT ( 'NONE',  ( -11.24178095869206828, 4.999999999999999112, 1.000000000000000000 ) ) ;
#4435=FACE_OUTER_BOUND ( 'NONE', #10331, .T. ) ;
#4438=VERTEX_POINT ( 'NONE', #2540 ) ;
#4445=ORIENTED_EDGE ( 'NONE', *, *, #4514, .F. ) ;
#4447=CARTESIAN_POINT ( 'NONE',  ( 0.000000000000000000, 4.999999999999999112, 1.000000000000000000 ) ) ;
#4449=VERTEX_POINT ( 'NONE', #12167 ) ;
#4450=VECTOR ( 'NONE', #13495, 1000.000000000000000 ) ;
#4452=ORIENTED_EDGE ( 'NONE', *, *, #18497, .F. ) ;
#4455=EDGE_LOOP ( 'NONE', ( #19066, #3829, #8075, #8869 ) ) ;
#4458=FACE_OUTER_BOUND ( 'NONE', #8775, .T. ) ;
#4460=CARTESIAN_POINT ( 'NONE',  ( -19.48630159782011262, 4.999999999999999112, 1.000000000000000000 ) ) ;
#4463=CARTESIAN_POINT ( 'NONE',  ( 0.000000000000000000, 9.000000000000001776, 1.000000000000000000 ) ) ;
#4469=EDGE_CURVE ( 'NONE', #5740, #7202, #9236, .T. ) ;
#4475=DIRECTION ( 'NONE',  ( 1.000000000000000000, 0.000000000000000000, 0.000000000000000000 ) ) ;
#4479=ORIENTED_EDGE ( 'NONE', *, *, #11903, .T. ) ;
#4485=DIRECTION ( 'NONE',  ( 0.000000000000000000, 1.000000000000000000, -0.000000000000000000 ) ) ;
#4498=LINE ( 'NONE', #17151, #8234 ) ;
#4502=ADVANCED_FACE ( 'NONE', ( #1092 ), #13731, .T. ) ;
#4505=FACE_OUTER_BOUND ( 'NONE', #19271, .T. ) ;
#4506=CARTESIAN_POINT ( 'NONE',  ( 25.04469207716615031, 4.999999999999999112, 0.000000000000000000 ) ) ;
#4514=EDGE_CURVE ( 'NONE', #7075, #5681, #15200, .T. ) ;
#4521=VERTEX_POINT ( 'NONE', #2441 ) ;
#4527=ADVANCED_FACE ( 'NONE', ( #10817 ), #15299, .T. ) ;
#4528=LINE ( 'NONE', #16137, #4388 ) ;
#4540=ORIENTED_EDGE ( 'NONE', *, *, #448, .F. ) ;
#4543=DIRECTION ( 'NONE',  ( 0.000000000000000000, 1.000000000000000000, 0.000000000000000000 ) ) ;
#4547=DIRECTION ( 'NONE',  ( 0.000000000000000000, 1.000000000000000000, -0.000000000000000000 ) ) ;
#4548=ORIENTED_EDGE ( 'NONE', *, *, #174, .F. ) ;
#4560=CARTESIAN_POINT ( 'NONE',  ( 17.30017143803810242, 0.000000000000000000, 1.000000000000000000 ) ) ;
#4565=EDGE_LOOP ( 'NONE', ( #2551, #17946, #2660, #8051, #10413, #15479, #2556, #15901, #16681, #14107, #18364, #4132, #8765, #19552, #20439, #8772, #707, #14031, #14827, #15809, #19870, #12680, #582, #14440, #6785, #4610, #9110, #15762, #15213, #3157, #11006, #12841, #10328, #17635, #15904, #7765, #9075, #8130, #940, #9839, #16813, #12721, #5053, #8416, #984, #2507, #18132, #19871, #12586, #6552, #1815, #6968, #7689, #4287, #820, #5910, #2398, #3358, #14949, #6127, #1670, #17920, #5839, #15957, #8603, #5384, #7574, #3409, #7579, #2852, #19350, #19861, #17351, #91, #20149, #9329, #8176, #5211, #1751, #12786, #6009, #3534, #1540, #11108, #5493, #5091, #18646, #14009, #9406, #13160, #11166, #16785, #13231, #7485, #8528, #6682, #126, #13904, #11379, #16962, #20636, #12556, #16675, #11375, #3257, #3925, #14301, #16477, #7864, #121, #10126, #10129, #8938, #3899, #8318, #6215, #18209, #15122, #4548, #5235, #17611, #305, #13384, #18492 ) ) ;
#4570=DIRECTION ( 'NONE',  ( 0.000000000000000000, 1.000000000000000000, 0.000000000000000000 ) ) ;
#4573=EDGE_LOOP ( 'NONE', ( #7624, #4138, #18621, #13413 ) ) ;
#4584=ORIENTED_EDGE ( 'NONE', *, *, #16503, .T. ) ;
#4588=CARTESIAN_POINT ( 'NONE',  ( 11.99178095869207006, 4.999999999999999112, 0.000000000000000000 ) ) ;
#4594=VERTEX_POINT ( 'NONE', #10599 ) ;
#4597=DIRECTION ( 'NONE',  ( -0.000000000000000000, -0.000000000000000000, -1.000000000000000000 ) ) ;
#4601=DIRECTION ( 'NONE',  ( 0.000000000000000000, 1.000000000000000000, 0.000000000000000000 ) ) ;
#4605=DIRECTION ( 'NONE',  ( 1.000000000000000000, 0.000000000000000000, 0.000000000000000000 ) ) ;
#4610=ORIENTED_EDGE ( 'NONE', *, *, #14523, .F. ) ;
#4630=EDGE_CURVE ( 'NONE', #9608, #10392, #12373, .T. ) ;
#4631=VERTEX_POINT ( 'NONE', #14558 ) ;
#4640=LINE ( 'NONE', #6011, #17395 ) ;
#4641=LINE ( 'NONE', #148, #16024 ) ;
#4644=LINE ( 'NONE', #20566, #18127 ) ;
#4648=DIRECTION ( 'NONE',  ( -0.000000000000000000, -0.000000000000000000, -1.000000000000000000 ) ) ;
#4649=EDGE_CURVE ( 'NONE', #14875, #17347, #8192, .T. ) ;
#4656=AXIS2_PLACEMENT_3D ( 'NONE', #17016, #1721, #17503 ) ;
#4660=VECTOR ( 'NONE', #10945, 1000.000000000000000 ) ;
#4676=DIRECTION ( 'NONE',  ( 0.000000000000000000, 0.000000000000000000, 1.000000000000000000 ) ) ;
#4678=EDGE_CURVE ( 'NONE', #14879, #19147, #137, .T. ) ;
#4680=CARTESIAN_POINT ( 'NONE',  ( 23.10856191738414012, 0.000000000000000000, 0.000000000000000000 ) ) ;
#4682=AXIS2_PLACEMENT_3D ( 'NONE', #8423, #19517, #16657 ) ;
#4692=EDGE_LOOP ( 'NONE', ( #6173, #5109, #5987, #15010 ) ) ;
#4693=ADVANCED_FACE ( 'NONE', ( #12783 ), #3269, .T. ) ;
#4695=CARTESIAN_POINT ( 'NONE',  ( 13.42791111847407848, 0.000000000000000000, 1.000000000000000000 ) ) ;
#4697=VERTEX_POINT ( 'NONE', #9645 ) ;
#4700=DIRECTION ( 'NONE',  ( -0.000000000000000000, -0.000000000000000000, -1.000000000000000000 ) ) ;
#4703=DIRECTION ( 'NONE',  ( 0.000000000000000000, -1.000000000000000000, 0.000000000000000000 ) ) ;
#4704=VECTOR ( 'NONE', #1272, 1000.000000000000000 ) ;
#4707=VECTOR ( 'NONE', #8845, 1000.000000000000000 ) ;
#4708=VECTOR ( 'NONE', #3707, 1000.000000000000000 ) ;
#4709=VECTOR ( 'NONE', #16028, 1000.000000000000000 ) ;
#4710=LINE ( 'NONE', #19776, #11035 ) ;
#4714=LINE ( 'NONE', #10998, #19436 ) ;
#4715=FACE_OUTER_BOUND ( 'NONE', #2927, .T. ) ;
#4716=EDGE_CURVE ( 'NONE', #1688, #12251, #15818, .T. ) ;
#4719=ORIENTED_EDGE ( 'NONE', *, *, #5705, .F. ) ;
#4724=VECTOR ( 'NONE', #6752, 999.9999999999998863 ) ;
#4725=ORIENTED_EDGE ( 'NONE', *, *, #15911, .T. ) ;
#4736=AXIS2_PLACEMENT_3D ( 'NONE', #20708, #15776, #18828 ) ;
#4739=VERTEX_POINT ( 'NONE', #2962 ) ;
#4746=CARTESIAN_POINT ( 'NONE',  ( 0.000000000000000000, 9.000000000000001776, 0.000000000000000000 ) ) ;
#4749=EDGE_CURVE ( 'NONE', #14732, #17662, #7058, .T. ) ;
#4751=CARTESIAN_POINT ( 'NONE',  ( -5.999999999999999112, -7.500000000000047073, 2.000000000000000000 ) ) ;
#4755=EDGE_CURVE ( 'NONE', #18278, #3865, #18870, .T. ) ;
#4763=LINE ( 'NONE', #3198, #7970 ) ;
#4769=VECTOR ( 'NONE', #14335, 1000.000000000000000 ) ;
#4771=ORIENTED_EDGE ( 'NONE', *, *, #11475, .F. ) ;
#4773=LINE ( 'NONE', #19624, #2358 ) ;
#4780=VERTEX_POINT ( 'NONE', #3376 ) ;
#4790=( LENGTH_UNIT ( ) NAMED_UNIT ( * ) SI_UNIT ( .MILLI., .METRE. ) );
#4796=CARTESIAN_POINT ( 'NONE',  ( -3.997260319564023501, 9.000000000000001776, 0.000000000000000000 ) ) ;
#4798=ORIENTED_EDGE ( 'NONE', *, *, #4350, .F. ) ;
#4816=CARTESIAN_POINT ( 'NONE',  ( -26.04469207716614676, 4.999999999999999112, 1.000000000000000000 ) ) ;
#4820=LINE ( 'NONE', #6089, #17067 ) ;
#4830=CARTESIAN_POINT ( 'NONE',  ( 17.30017143803810242, 4.999999999999999112, 1.000000000000000000 ) ) ;
#4831=DIRECTION ( 'NONE',  ( 1.000000000000000000, 0.000000000000000000, -0.000000000000000000 ) ) ;
#4832=CARTESIAN_POINT ( 'NONE',  ( 4.999999999999998224, -7.500000000000047073, 9.999999999999998224 ) ) ;
#4834=CARTESIAN_POINT ( 'NONE',  ( 0.000000000000000000, 4.999999999999999112, 1.000000000000000000 ) ) ;
#4839=DIRECTION ( 'NONE',  ( -0.000000000000000000, -0.000000000000000000, -1.000000000000000000 ) ) ;
#4847=VERTEX_POINT ( 'NONE', #10068 ) ;
#4850=CARTESIAN_POINT ( 'NONE',  ( 8.119520639128047890, 0.000000000000000000, 1.000000000000000000 ) ) ;
#4851=VERTEX_POINT ( 'NONE', #14663 ) ;
#4853=CARTESIAN_POINT ( 'NONE',  ( -5.933390479346035029, 4.999999999999999112, 1.000000000000000000 ) ) ;
#4854=COLOUR_RGB ( '', 0.09019608, 0.27058824, 0.51372549) ;
#4857=DIRECTION ( 'NONE',  ( 1.000000000000000000, 0.000000000000000000, 0.000000000000000000 ) ) ;
#4862=LINE ( 'NONE', #12707, #6016 ) ;
#4866=VECTOR ( 'NONE', #11989, 1000.000000000000000 ) ;
#4872=EDGE_CURVE ( 'NONE', #11469, #18418, #2313, .T. ) ;
#4874=VERTEX_POINT ( 'NONE', #14769 ) ;
#4886=EDGE_CURVE ( 'NONE', #8434, #16176, #13401, .T. ) ;
#4890=ORIENTED_EDGE ( 'NONE', *, *, #15799, .T. ) ;
#4892=EDGE_CURVE ( 'NONE', #9041, #10100, #9954, .T. ) ;
#4893=PLANE ( 'NONE',  #4736 ) ;
#4898=CARTESIAN_POINT ( 'NONE',  ( -13.67791111847408025, 9.000000000000001776, 1.000000000000000000 ) ) ;
#4907=DIRECTION ( 'NONE',  ( -0.000000000000000000, -0.000000000000000000, -1.000000000000000000 ) ) ;
#4912=EDGE_CURVE ( 'NONE', #14572, #13516, #5149, .T. ) ;
#4922=ORIENTED_EDGE ( 'NONE', *, *, #6382, .T. ) ;
#4923=ORIENTED_EDGE ( 'NONE', *, *, #9382, .T. ) ;
#4925=AXIS2_PLACEMENT_3D ( 'NONE', #11285, #6270, #15687 ) ;
#4927=LINE ( 'NONE', #328, #9348 ) ;
#4930=CARTESIAN_POINT ( 'NONE',  ( -5.933390479346035029, 4.999999999999999112, 0.000000000000000000 ) ) ;
#4931=DIRECTION ( 'NONE',  ( -1.000000000000000000, 0.000000000000000000, -0.000000000000000000 ) ) ;
#4936=EDGE_CURVE ( 'NONE', #11456, #9694, #11623, .T. ) ;
#4939=DIRECTION ( 'NONE',  ( -0.000000000000000000, -0.000000000000000000, -1.000000000000000000 ) ) ;
#4949=ORIENTED_EDGE ( 'NONE', *, *, #6104, .T. ) ;
#4952=CARTESIAN_POINT ( 'NONE',  ( -3.997260319564023501, 9.000000000000001776, 1.000000000000000000 ) ) ;
#4954=EDGE_CURVE ( 'NONE', #8157, #7916, #8498, .T. ) ;
#4956=DIRECTION ( 'NONE',  ( 1.000000000000000000, 0.000000000000000000, 0.000000000000000000 ) ) ;
#4958=CARTESIAN_POINT ( 'NONE',  ( -24.79469207716615031, 9.000000000000001776, 1.000000000000000000 ) ) ;
#4963=CARTESIAN_POINT ( 'NONE',  ( -25.29469207716615031, 0.000000000000000000, 1.000000000000000000 ) ) ;
#4964=DIRECTION ( 'NONE',  ( -0.000000000000000000, -0.000000000000000000, -1.000000000000000000 ) ) ;
#4966=CARTESIAN_POINT ( 'NONE',  ( -7.869520639128047002, 4.999999999999999112, 1.000000000000000000 ) ) ;
#4975=VERTEX_POINT ( 'NONE', #8595 ) ;
#4978=ORIENTED_EDGE ( 'NONE', *, *, #13856, .T. ) ;
#4979=VERTEX_POINT ( 'NONE', #646 ) ;
#4981=VERTEX_POINT ( 'NONE', #543 ) ;
#4983=EDGE_CURVE ( 'NONE', #8074, #999, #18224, .T. ) ;
#4984=VECTOR ( 'NONE', #4857, 1000.000000000000000 ) ;
#4987=DIRECTION ( 'NONE',  ( -0.000000000000000000, -0.000000000000000000, -1.000000000000000000 ) ) ;
#4989=CARTESIAN_POINT ( 'NONE',  ( -25.29469207716615031, 9.000000000000001776, 1.000000000000000000 ) ) ;
#4991=DIRECTION ( 'NONE',  ( 1.000000000000000000, 0.000000000000000000, 0.000000000000000000 ) ) ;
#5000=ORIENTED_EDGE ( 'NONE', *, *, #2432, .T. ) ;
#5002=FACE_OUTER_BOUND ( 'NONE', #7682, .T. ) ;
#5004=ORIENTED_EDGE ( 'NONE', *, *, #11635, .T. ) ;
#5007=VERTEX_POINT ( 'NONE', #954 ) ;
#5009=EDGE_CURVE ( 'NONE', #5007, #16377, #13811, .T. ) ;
#5011=EDGE_LOOP ( 'NONE', ( #7940, #8254, #7686, #4923 ) ) ;
#5013=FACE_OUTER_BOUND ( 'NONE', #18208, .T. ) ;
#5018=LINE ( 'NONE', #18196, #14021 ) ;
#5028=ORIENTED_EDGE ( 'NONE', *, *, #6218, .T. ) ;
#5029=VERTEX_POINT ( 'NONE', #12040 ) ;
#5031=CARTESIAN_POINT ( 'NONE',  ( 13.92791111847407848, 4.999999999999999112, 0.000000000000000000 ) ) ;
#5034=EDGE_CURVE ( 'NONE', #17531, #16862, #10795, .T. ) ;
#5038=CIRCLE ( 'NONE', #11701, 0.4999999999999987232 ) ;
#5043=VECTOR ( 'NONE', #7031, 1000.000000000000000 ) ;
#5044=FACE_OUTER_BOUND ( 'NONE', #5011, .T. ) ;
#5053=ORIENTED_EDGE ( 'NONE', *, *, #17145, .F. ) ;
#5056=VECTOR ( 'NONE', #19827, 1000.000000000000000 ) ;
#5063=ORIENTED_EDGE ( 'NONE', *, *, #10818, .T. ) ;
#5066=ADVANCED_FACE ( 'NONE', ( #18326 ), #7448, .T. ) ;
#5067=LINE ( 'NONE', #11138, #19463 ) ;
#5069=DIRECTION ( 'NONE',  ( 1.000000000000000000, 0.000000000000000000, 0.000000000000000000 ) ) ;
#5074=DIRECTION ( 'NONE',  ( 0.000000000000000000, -1.000000000000000000, 0.000000000000000000 ) ) ;
#5076=FACE_OUTER_BOUND ( 'NONE', #2272, .T. ) ;
#5078=DIRECTION ( 'NONE',  ( 1.000000000000000000, 0.000000000000000000, 0.000000000000000000 ) ) ;
#5084=ORIENTED_EDGE ( 'NONE', *, *, #7502, .T. ) ;
#5090=DIRECTION ( 'NONE',  ( 0.000000000000000000, -1.000000000000000000, 0.000000000000000000 ) ) ;
#5091=ORIENTED_EDGE ( 'NONE', *, *, #5357, .F. ) ;
#5095=CARTESIAN_POINT ( 'NONE',  ( 10.05565079891005631, 9.000000000000001776, 0.000000000000000000 ) ) ;
#5097=DIRECTION ( 'NONE',  ( 1.000000000000000000, 0.000000000000000000, 0.000000000000000000 ) ) ;
#5099=VECTOR ( 'NONE', #19379, 1000.000000000000000 ) ;
#5105=ORIENTED_EDGE ( 'NONE', *, *, #11297, .F. ) ;
#5109=ORIENTED_EDGE ( 'NONE', *, *, #3340, .F. ) ;
#5110=LINE ( 'NONE', #11587, #2269 ) ;
#5111=CARTESIAN_POINT ( 'NONE',  ( 0.000000000000000000, 4.999999999999999112, 1.000000000000000000 ) ) ;
#5112=VECTOR ( 'NONE', #18920, 1000.000000000000000 ) ;
#5113=ORIENTED_EDGE ( 'NONE', *, *, #12618, .F. ) ;
#5114=ORIENTED_EDGE ( 'NONE', *, *, #3747, .T. ) ;
#5117=EDGE_LOOP ( 'NONE', ( #2770, #14549, #1257, #6077 ) ) ;
#5120=FACE_OUTER_BOUND ( 'NONE', #8997, .T. ) ;
#5128=ADVANCED_FACE ( 'NONE', ( #4715 ), #11104, .T. ) ;
#5138=CARTESIAN_POINT ( 'NONE',  ( -18.98630159782011262, 9.000000000000001776, 1.000000000000000000 ) ) ;
#5142=DIRECTION ( 'NONE',  ( 0.000000000000000000, -0.000000000000000000, -1.000000000000000000 ) ) ;
#5149=LINE ( 'NONE', #231, #18426 ) ;
#5157=VERTEX_POINT ( 'NONE', #14846 ) ;
#5160=CARTESIAN_POINT ( 'NONE',  ( 26.79469207716614676, 9.000000000000001776, 1.000000000000000000 ) ) ;
#5161=ORIENTED_EDGE ( 'NONE', *, *, #8129, .T. ) ;
#5164=FACE_OUTER_BOUND ( 'NONE', #16366, .T. ) ;
#5169=FACE_OUTER_BOUND ( 'NONE', #18832, .T. ) ;
#5172=DIRECTION ( 'NONE',  ( -1.000000000000000000, -1.013672804646636192E-16, 0.000000000000000000 ) ) ;
#5176=ORIENTED_EDGE ( 'NONE', *, *, #174, .T. ) ;
#5181=ORIENTED_EDGE ( 'NONE', *, *, #11019, .T. ) ;
#5184=DIRECTION ( 'NONE',  ( -1.000000000000000000, 0.000000000000000000, 0.000000000000000000 ) ) ;
#5187=DIRECTION ( 'NONE',  ( 0.000000000000000000, 1.000000000000000000, 0.000000000000000000 ) ) ;
#5190=VECTOR ( 'NONE', #15940, 1000.000000000000000 ) ;
#5192=CARTESIAN_POINT ( 'NONE',  ( 4.247260319564023945, 4.999999999999999112, 1.000000000000000000 ) ) ;
#5194=PLANE ( 'NONE',  #11979 ) ;
#5197=VECTOR ( 'NONE', #11017, 1000.000000000000000 ) ;
#5199=EDGE_CURVE ( 'NONE', #3720, #9059, #14749, .T. ) ;
#5207=ORIENTED_EDGE ( 'NONE', *, *, #18074, .F. ) ;
#5208=LINE ( 'NONE', #14829, #4272 ) ;
#5211=ORIENTED_EDGE ( 'NONE', *, *, #2333, .F. ) ;
#5217=CARTESIAN_POINT ( 'NONE',  ( -27.50000000000000711, 4.999999999999999112, 1.000000000000000000 ) ) ;
#5235=ORIENTED_EDGE ( 'NONE', *, *, #1486, .F. ) ;
#5236=CARTESIAN_POINT ( 'NONE',  ( 13.92791111847407848, 4.999999999999999112, 1.000000000000000000 ) ) ;
#5238=CARTESIAN_POINT ( 'NONE',  ( -24.79469207716615031, 0.000000000000000000, 1.000000000000000000 ) ) ;
#5256=VECTOR ( 'NONE', #17352, 1000.000000000000000 ) ;
#5259=VERTEX_POINT ( 'NONE', #10045 ) ;
#5269=LINE ( 'NONE', #14888, #9062 ) ;
#5270=AXIS2_PLACEMENT_3D ( 'NONE', #4058, #7512, #18498 ) ;
#5271=AXIS2_PLACEMENT_3D ( 'NONE', #2784, #8853, #5916 ) ;
#5284=ORIENTED_EDGE ( 'NONE', *, *, #12509, .F. ) ;
#5285=DIRECTION ( 'NONE',  ( 0.4999999999999948930, 0.8660254037844415942, -0.000000000000000000 ) ) ;
#5287=DIRECTION ( 'NONE',  ( 0.000000000000000000, -1.000000000000000000, 0.000000000000000000 ) ) ;
#5289=VERTEX_POINT ( 'NONE', #6805 ) ;
#5298=VECTOR ( 'NONE', #2701, 1000.000000000000000 ) ;
#5300=DIRECTION ( 'NONE',  ( 0.000000000000000000, -1.000000000000000000, 0.000000000000000000 ) ) ;
#5307=ORIENTED_EDGE ( 'NONE', *, *, #12271, .F. ) ;
#5316=AXIS2_PLACEMENT_3D ( 'NONE', #15367, #17456, #18727 ) ;
#5327=VECTOR ( 'NONE', #18478, 1000.000000000000000 ) ;
#5333=CARTESIAN_POINT ( 'NONE',  ( -23.35856191738413656, 9.000000000000001776, 0.000000000000000000 ) ) ;
#5335=VECTOR ( 'NONE', #13372, 1000.000000000000000 ) ;
#5338=ORIENTED_EDGE ( 'NONE', *, *, #6586, .F. ) ;
#5339=ORIENTED_EDGE ( 'NONE', *, *, #7162, .T. ) ;
#5344=CARTESIAN_POINT ( 'NONE',  ( -5.999999999999999112, -2.500000000000047518, 2.000000000000000000 ) ) ;
#5345=FACE_OUTER_BOUND ( 'NONE', #18911, .T. ) ;
#5349=LINE ( 'NONE', #13700, #7857 ) ;
#5357=EDGE_CURVE ( 'NONE', #9608, #11456, #19885, .T. ) ;
#5366=VECTOR ( 'NONE', #5807, 1000.000000000000000 ) ;
#5367=VERTEX_POINT ( 'NONE', #10462 ) ;
#5368=VECTOR ( 'NONE', #9571, 1000.000000000000000 ) ;
#5379=FACE_OUTER_BOUND ( 'NONE', #1336, .T. ) ;
#5384=ORIENTED_EDGE ( 'NONE', *, *, #12459, .F. ) ;
#5392=ORIENTED_EDGE ( 'NONE', *, *, #7241, .T. ) ;
#5395=VERTEX_POINT ( 'NONE', #15257 ) ;
#5398=EDGE_CURVE ( 'NONE', #122, #7075, #4278, .T. ) ;
#5399=VECTOR ( 'NONE', #12884, 1000.000000000000000 ) ;
#5418=FACE_OUTER_BOUND ( 'NONE', #14110, .T. ) ;
#5422=VECTOR ( 'NONE', #19579, 1000.000000000000000 ) ;
#5438=EDGE_CURVE ( 'NONE', #4739, #13902, #8991, .T. ) ;
#5441=CARTESIAN_POINT ( 'NONE',  ( -4.174178364069194536E-16, 3.500000000000001332, 1.000000000000000000 ) ) ;
#5443=VECTOR ( 'NONE', #769, 1000.000000000000000 ) ;
#5445=DIRECTION ( 'NONE',  ( 1.000000000000000000, 0.000000000000000000, 0.000000000000000000 ) ) ;
#5446=ORIENTED_EDGE ( 'NONE', *, *, #19002, .T. ) ;
#5451=CARTESIAN_POINT ( 'NONE',  ( -3.997260319564023501, 9.000000000000001776, 1.000000000000000000 ) ) ;
#5456=CARTESIAN_POINT ( 'NONE',  ( -17.55017143803810242, 4.999999999999999112, 1.000000000000000000 ) ) ;
#5462=CARTESIAN_POINT ( 'NONE',  ( 0.000000000000000000, 4.999999999999999112, 1.000000000000000000 ) ) ;
#5468=ORIENTED_EDGE ( 'NONE', *, *, #8876, .T. ) ;
#5490=VERTEX_POINT ( 'NONE', #17141 ) ;
#5492=LINE ( 'NONE', #16784, #4707 ) ;
#5493=ORIENTED_EDGE ( 'NONE', *, *, #4936, .F. ) ;
#5494=VERTEX_POINT ( 'NONE', #16930 ) ;
#5508=VECTOR ( 'NONE', #9210, 1000.000000000000000 ) ;
#5514=ORIENTED_EDGE ( 'NONE', *, *, #6104, .F. ) ;
#5519=CARTESIAN_POINT ( 'NONE',  ( 5.999999999999999112, -7.500000000000047073, 2.000000000000000000 ) ) ;
#5520=CARTESIAN_POINT ( 'NONE',  ( -7.869520639128047002, 9.000000000000001776, 1.000000000000000000 ) ) ;
#5525=ORIENTED_EDGE ( 'NONE', *, *, #15152, .T. ) ;
#5539=ORIENTED_EDGE ( 'NONE', *, *, #1802, .T. ) ;
#5546=EDGE_LOOP ( 'NONE', ( #14357, #19986, #7203, #16280, #17408, #20074, #4949, #18567, #2695, #14752, #16809, #1697 ) ) ;
#5550=VERTEX_POINT ( 'NONE', #18414 ) ;
#5552=DIRECTION ( 'NONE',  ( 0.000000000000000000, -1.000000000000000000, 0.000000000000000000 ) ) ;
#5553=PLANE ( 'NONE',  #11971 ) ;
#5555=EDGE_CURVE ( 'NONE', #20689, #14130, #16831, .T. ) ;
#5556=CARTESIAN_POINT ( 'NONE',  ( -23.35856191738413656, 0.000000000000000000, 1.000000000000000000 ) ) ;
#5560=DIRECTION ( 'NONE',  ( 0.000000000000000000, -0.000000000000000000, 1.000000000000000000 ) ) ;
#5563=CARTESIAN_POINT ( 'NONE',  ( 3.747260319564023501, 9.000000000000001776, 1.000000000000000000 ) ) ;
#5565=EDGE_CURVE ( 'NONE', #5007, #485, #1251, .T. ) ;
#5573=VERTEX_POINT ( 'NONE', #10974 ) ;
#5576=CARTESIAN_POINT ( 'NONE',  ( 0.000000000000000000, 9.000000000000001776, 0.000000000000000000 ) ) ;
#5578=ADVANCED_FACE ( 'NONE', ( #10876 ), #14409, .F. ) ;
#5582=FACE_OUTER_BOUND ( 'NONE', #15165, .T. ) ;
#5583=AXIS2_PLACEMENT_3D ( 'NONE', #12031, #10889, #12139 ) ;
#5586=CARTESIAN_POINT ( 'NONE',  ( 0.000000000000000000, 4.999999999999999112, 1.000000000000000000 ) ) ;
#5598=ORIENTED_EDGE ( 'NONE', *, *, #14003, .T. ) ;
#5599=ORIENTED_EDGE ( 'NONE', *, *, #2749, .F. ) ;
#5600=DIRECTION ( 'NONE',  ( 0.000000000000000000, -0.000000000000000000, 1.000000000000000000 ) ) ;
#5601=ORIENTED_EDGE ( 'NONE', *, *, #6527, .F. ) ;
#5606=DIRECTION ( 'NONE',  ( 0.000000000000000000, -1.000000000000000000, 0.000000000000000000 ) ) ;
#5615=EDGE_CURVE ( 'NONE', #20251, #17893, #3227, .T. ) ;
#5621=ORIENTED_EDGE ( 'NONE', *, *, #15464, .T. ) ;
#5630=LINE ( 'NONE', #4065, #3592 ) ;
#5631=VECTOR ( 'NONE', #12030, 1000.000000000000000 ) ;
#5646=EDGE_CURVE ( 'NONE', #14589, #11516, #9598, .T. ) ;
#5648=CARTESIAN_POINT ( 'NONE',  ( 0.000000000000000000, 9.000000000000001776, 0.000000000000000000 ) ) ;
#5653=DIRECTION ( 'NONE',  ( 1.000000000000000000, 0.000000000000000000, 0.000000000000000000 ) ) ;
#5655=EDGE_LOOP ( 'NONE', ( #8768, #3467, #13427, #14466 ) ) ;
#5656=CARTESIAN_POINT ( 'NONE',  ( -7.369520639128046113, 0.000000000000000000, 0.000000000000000000 ) ) ;
#5659=CARTESIAN_POINT ( 'NONE',  ( -5.433390479346035029, 4.999999999999999112, 1.000000000000000000 ) ) ;
#5661=CARTESIAN_POINT ( 'NONE',  ( -13.00000000000000355, 0.000000000000000000, 1.000000000000000000 ) ) ;
#5671=CARTESIAN_POINT ( 'NONE',  ( 23.10856191738414012, 4.999999999999999112, 1.000000000000000000 ) ) ;
#5680=DIRECTION ( 'NONE',  ( 0.000000000000000000, 1.000000000000000000, 0.000000000000000000 ) ) ;
#5681=VERTEX_POINT ( 'NONE', #4796 ) ;
#5690=CARTESIAN_POINT ( 'NONE',  ( 0.000000000000000000, 9.000000000000000000, 1.000000000000000000 ) ) ;
#5696=EDGE_LOOP ( 'NONE', ( #19728, #5782, #6765, #6254 ) ) ;
#5697=AXIS2_PLACEMENT_3D ( 'NONE', #7347, #20216, #19910 ) ;
#5700=CIRCLE ( 'NONE', #18725, 2.999999999999999112 ) ;
#5705=EDGE_CURVE ( 'NONE', #16350, #6813, #1551, .T. ) ;
#5708=ORIENTED_EDGE ( 'NONE', *, *, #14971, .F. ) ;
#5709=ORIENTED_EDGE ( 'NONE', *, *, #3165, .F. ) ;
#5714=AXIS2_PLACEMENT_3D ( 'NONE', #8743, #1105, #7483 ) ;
#5716=ADVANCED_FACE ( 'NONE', ( #15976 ), #4893, .T. ) ;
#5718=VECTOR ( 'NONE', #6845, 1000.000000000000000 ) ;
#5725=CARTESIAN_POINT ( 'NONE',  ( 26.04469207716615031, 0.000000000000000000, 0.000000000000000000 ) ) ;
#5735=VERTEX_POINT ( 'NONE', #1456 ) ;
#5739=ORIENTED_EDGE ( 'NONE', *, *, #11586, .F. ) ;
#5740=VERTEX_POINT ( 'NONE', #7835 ) ;
#5741=ORIENTED_EDGE ( 'NONE', *, *, #17813, .F. ) ;
#5742=CARTESIAN_POINT ( 'NONE',  ( 20.00000000000000000, -5.999999999999994671, 1.000000000000000000 ) ) ;
#5744=DIRECTION ( 'NONE',  ( -1.000000000000000000, 0.000000000000000000, 0.000000000000000000 ) ) ;
#5746=CARTESIAN_POINT ( 'NONE',  ( 25.54469207716615031, 0.000000000000000000, 1.000000000000000000 ) ) ;
#5747=LINE ( 'NONE', #1449, #18093 ) ;
#5754=LINE ( 'NONE', #8989, #3945 ) ;
#5759=ORIENTED_EDGE ( 'NONE', *, *, #4302, .T. ) ;
#5763=ORIENTED_EDGE ( 'NONE', *, *, #14331, .T. ) ;
#5766=PLANE ( 'NONE',  #16708 ) ;
#5768=LINE ( 'NONE', #7641, #18282 ) ;
#5774=CARTESIAN_POINT ( 'NONE',  ( 0.000000000000000000, 4.999999999999999112, 1.000000000000000000 ) ) ;
#5782=ORIENTED_EDGE ( 'NONE', *, *, #4200, .F. ) ;
#5784=CARTESIAN_POINT ( 'NONE',  ( -7.369520639128046113, 4.999999999999999112, 0.000000000000000000 ) ) ;
#5788=VECTOR ( 'NONE', #15988, 1000.000000000000000 ) ;
#5792=ADVANCED_FACE ( 'NONE', ( #7700 ), #617, .T. ) ;
#5795=LINE ( 'NONE', #9235, #10838 ) ;
#5802=DIRECTION ( 'NONE',  ( -0.000000000000000000, -0.000000000000000000, -1.000000000000000000 ) ) ;
#5807=DIRECTION ( 'NONE',  ( 1.000000000000000000, 0.000000000000000000, 0.000000000000000000 ) ) ;
#5809=EDGE_CURVE ( 'NONE', #12435, #4874, #2789, .T. ) ;
#5812=ORIENTED_EDGE ( 'NONE', *, *, #15869, .F. ) ;
#5814=VECTOR ( 'NONE', #8832, 1000.000000000000000 ) ;
#5817=CARTESIAN_POINT ( 'NONE',  ( -27.49999999999999645, -4.770489558936219510E-14, 0.000000000000000000 ) ) ;
#5819=EDGE_CURVE ( 'NONE', #15395, #3029, #19775, .T. ) ;
#5820=ADVANCED_FACE ( 'NONE', ( #3860 ), #8783, .T. ) ;
#5832=ORIENTED_EDGE ( 'NONE', *, *, #6586, .T. ) ;
#5838=DIRECTION ( 'NONE',  ( 1.000000000000000000, 0.000000000000000000, -0.000000000000000000 ) ) ;
#5839=ORIENTED_EDGE ( 'NONE', *, *, #2732, .F. ) ;
#5845=EDGE_CURVE ( 'NONE', #14133, #13753, #1220, .T. ) ;
#5848=LINE ( 'NONE', #12732, #2691 ) ;
#5854=ORIENTED_EDGE ( 'NONE', *, *, #4678, .T. ) ;
#5858=EDGE_CURVE ( 'NONE', #7250, #13818, #9368, .T. ) ;
#5860=DIRECTION ( 'NONE',  ( -1.000000000000000000, 0.000000000000000000, 0.000000000000000000 ) ) ;
#5862=ORIENTED_EDGE ( 'NONE', *, *, #7858, .F. ) ;
#5867=ORIENTED_EDGE ( 'NONE', *, *, #1874, .F. ) ;
#5872=DIRECTION ( 'NONE',  ( 0.000000000000000000, 1.000000000000000000, -0.000000000000000000 ) ) ;
#5874=VECTOR ( 'NONE', #17221, 1000.000000000000000 ) ;
#5881=ORIENTED_EDGE ( 'NONE', *, *, #1798, .F. ) ;
#5885=EDGE_CURVE ( 'NONE', #610, #2607, #14168, .T. ) ;
#5891=CARTESIAN_POINT ( 'NONE',  ( 0.000000000000000000, 4.999999999999999112, 1.000000000000000000 ) ) ;
#5892=DIRECTION ( 'NONE',  ( 0.000000000000000000, -0.000000000000000000, 1.000000000000000000 ) ) ;
#5905=LINE ( 'NONE', #12584, #20422 ) ;
#5910=ORIENTED_EDGE ( 'NONE', *, *, #15898, .F. ) ;
#5912=CARTESIAN_POINT ( 'NONE',  ( -14.00147952833368770, -0.02431694168600004660, 0.6777495337877021964 ) ) ;
#5915=ORIENTED_EDGE ( 'NONE', *, *, #11787, .T. ) ;
#5916=DIRECTION ( 'NONE',  ( 0.000000000000000000, -0.000000000000000000, 1.000000000000000000 ) ) ;
#5918=CARTESIAN_POINT ( 'NONE',  ( -7.869520639128047002, 0.000000000000000000, 1.000000000000000000 ) ) ;
#5923=DIRECTION ( 'NONE',  ( 0.000000000000000000, -1.000000000000000000, 0.000000000000000000 ) ) ;
#5924=CARTESIAN_POINT ( 'NONE',  ( 15.36404127825609400, 9.000000000000001776, 0.000000000000000000 ) ) ;
#5963=VECTOR ( 'NONE', #15228, 1000.000000000000000 ) ;
#5964=CARTESIAN_POINT ( 'NONE',  ( -11.74178095869206828, 0.000000000000000000, 1.000000000000000000 ) ) ;
#5965=VECTOR ( 'NONE', #17002, 1000.000000000000000 ) ;
#5968=PLANE ( 'NONE',  #5583 ) ;
#5970=CARTESIAN_POINT ( 'NONE',  ( 20.00000000000000000, 3.000000000000004441, 1.000000000000000000 ) ) ;
#5978=VECTOR ( 'NONE', #11552, 1000.000000000000000 ) ;
#5979=DIRECTION ( 'NONE',  ( 0.000000000000000000, 0.000000000000000000, 1.000000000000000000 ) ) ;
#5983=ORIENTED_EDGE ( 'NONE', *, *, #19115, .T. ) ;
#5986=ORIENTED_EDGE ( 'NONE', *, *, #4238, .T. ) ;
#5987=ORIENTED_EDGE ( 'NONE', *, *, #1253, .T. ) ;
#5992=VECTOR ( 'NONE', #7099, 1000.000000000000000 ) ;
#6009=ORIENTED_EDGE ( 'NONE', *, *, #821, .F. ) ;
#6011=CARTESIAN_POINT ( 'NONE',  ( 21.67243175760212637, 0.000000000000000000, 0.000000000000000000 ) ) ;
#6012=VECTOR ( 'NONE', #9267, 1000.000000000000000 ) ;
#6015=DIRECTION ( 'NONE',  ( -0.000000000000000000, -0.000000000000000000, -1.000000000000000000 ) ) ;
#6016=VECTOR ( 'NONE', #6753, 1000.000000000000000 ) ;
#6023=VECTOR ( 'NONE', #17027, 1000.000000000000000 ) ;
#6025=LINE ( 'NONE', #13857, #7337 ) ;
#6027=DIRECTION ( 'NONE',  ( -0.000000000000000000, -0.000000000000000000, -1.000000000000000000 ) ) ;
#6039=EDGE_CURVE ( 'NONE', #9021, #9247, #9568, .T. ) ;
#6042=ORIENTED_EDGE ( 'NONE', *, *, #1798, .T. ) ;
#6048=VECTOR ( 'NONE', #1843, 1000.000000000000000 ) ;
#6050=VECTOR ( 'NONE', #16534, 1000.000000000000000 ) ;
#6051=VERTEX_POINT ( 'NONE', #14372 ) ;
#6053=PLANE ( 'NONE',  #10282 ) ;
#6055=PLANE ( 'NONE',  #14705 ) ;
#6057=EDGE_CURVE ( 'NONE', #18629, #12851, #11344, .T. ) ;
#6058=DIRECTION ( 'NONE',  ( -1.000000000000000000, 0.000000000000000000, 0.000000000000000000 ) ) ;
#6060=PRESENTATION_STYLE_ASSIGNMENT (( #1247 ) ) ;
#6067=ORIENTED_EDGE ( 'NONE', *, *, #3902, .F. ) ;
#6071=ORIENTED_EDGE ( 'NONE', *, *, #6527, .T. ) ;
#6073=CARTESIAN_POINT ( 'NONE',  ( 5.683390479346035029, 9.000000000000001776, 1.000000000000000000 ) ) ;
#6075=ADVANCED_FACE ( 'NONE', ( #11241 ), #12598, .T. ) ;
#6077=ORIENTED_EDGE ( 'NONE', *, *, #448, .T. ) ;
#6089=CARTESIAN_POINT ( 'NONE',  ( -13.17791111847408025, 4.999999999999999112, 1.000000000000000000 ) ) ;
#6091=VECTOR ( 'NONE', #16158, 1000.000000000000114 ) ;
#6096=FACE_OUTER_BOUND ( 'NONE', #4573, .T. ) ;
#6097=VERTEX_POINT ( 'NONE', #17636 ) ;
#6103=AXIS2_PLACEMENT_3D ( 'NONE', #2531, #18449, #16863 ) ;
#6104=EDGE_CURVE ( 'NONE', #15422, #49, #77, .T. ) ;
#6105=LINE ( 'NONE', #20331, #9388 ) ;
#6107=LINE ( 'NONE', #17595, #12360 ) ;
#6124=ORIENTED_EDGE ( 'NONE', *, *, #11640, .T. ) ;
#6127=ORIENTED_EDGE ( 'NONE', *, *, #6722, .F. ) ;
#6128=CARTESIAN_POINT ( 'NONE',  ( -24.50000000000000000, 0.000000000000000000, 1.000000000000000000 ) ) ;
#6129=CARTESIAN_POINT ( 'NONE',  ( 4.999999999999998224, -2.500000000000047518, 9.999999999999998224 ) ) ;
#6134=CARTESIAN_POINT ( 'NONE',  ( 3.999999999999999112, -7.500000000000047073, 9.999999999999998224 ) ) ;
#6136=DIRECTION ( 'NONE',  ( 0.000000000000000000, -1.000000000000000000, 0.000000000000000000 ) ) ;
#6149=VECTOR ( 'NONE', #15582, 1000.000000000000000 ) ;
#6157=CARTESIAN_POINT ( 'NONE',  ( -9.305650798910056309, 9.000000000000001776, 1.000000000000000000 ) ) ;
#6167=PLANE ( 'NONE',  #7325 ) ;
#6171=EDGE_CURVE ( 'NONE', #42, #7093, #16766, .T. ) ;
#6173=ORIENTED_EDGE ( 'NONE', *, *, #19115, .F. ) ;
#6176=ADVANCED_FACE ( 'NONE', ( #17751 ), #9897, .T. ) ;
#6180=CARTESIAN_POINT ( 'NONE',  ( 0.000000000000000000, 9.000000000000001776, 1.000000000000000000 ) ) ;
#6184=LINE ( 'NONE', #14323, #4704 ) ;
#6191=ORIENTED_EDGE ( 'NONE', *, *, #6746, .F. ) ;
#6192=ADVANCED_FACE ( 'NONE', ( #14281 ), #20690, .T. ) ;
#6194=CARTESIAN_POINT ( 'NONE',  ( 0.000000000000000000, 4.999999999999999112, 1.000000000000000000 ) ) ;
#6200=LINE ( 'NONE', #2959, #13539 ) ;
#6202=DIRECTION ( 'NONE',  ( -1.000000000000000000, 0.000000000000000000, 0.000000000000000000 ) ) ;
#6213=DIRECTION ( 'NONE',  ( 0.000000000000000000, -1.000000000000000000, 0.000000000000000000 ) ) ;
#6214=DIRECTION ( 'NONE',  ( -0.000000000000000000, -0.000000000000000000, -1.000000000000000000 ) ) ;
#6215=ORIENTED_EDGE ( 'NONE', *, *, #15799, .F. ) ;
#6217=ORIENTED_EDGE ( 'NONE', *, *, #4755, .F. ) ;
#6218=EDGE_CURVE ( 'NONE', #7096, #14361, #12722, .T. ) ;
#6219=LINE ( 'NONE', #14254, #10783 ) ;
#6220=CARTESIAN_POINT ( 'NONE',  ( -13.98883902916702482, -0.1144964390440934426, 0.8305393671244342135 ) ) ;
#6221=ORIENTED_EDGE ( 'NONE', *, *, #11418, .T. ) ;
#6222=LINE ( 'NONE', #6128, #12195 ) ;
#6226=CARTESIAN_POINT ( 'NONE',  ( 10.05565079891005631, 0.000000000000000000, 1.000000000000000000 ) ) ;
#6230=DIRECTION ( 'NONE',  ( -0.000000000000000000, -0.000000000000000000, -1.000000000000000000 ) ) ;
#6236=ORIENTED_EDGE ( 'NONE', *, *, #17554, .F. ) ;
#6239=VERTEX_POINT ( 'NONE', #1750 ) ;
#6241=EDGE_LOOP ( 'NONE', ( #5708, #1080, #10881, #4479 ) ) ;
#6245=PLANE ( 'NONE',  #3625 ) ;
#6249=ADVANCED_FACE ( 'NONE', ( #11163 ), #17534, .T. ) ;
#6254=ORIENTED_EDGE ( 'NONE', *, *, #17526, .T. ) ;
#6261=LINE ( 'NONE', #13897, #17332 ) ;
#6267=FACE_OUTER_BOUND ( 'NONE', #14777, .T. ) ;
#6270=DIRECTION ( 'NONE',  ( 0.000000000000000000, 1.000000000000000000, 0.000000000000000000 ) ) ;
#6273=AXIS2_PLACEMENT_3D ( 'NONE', #1968, #404, #19454 ) ;
#6275=DIRECTION ( 'NONE',  ( 1.000000000000000000, -0.000000000000000000, 0.000000000000000000 ) ) ;
#6279=EDGE_CURVE ( 'NONE', #15974, #19423, #14393, .T. ) ;
#6286=EDGE_CURVE ( 'NONE', #16176, #14054, #17947, .T. ) ;
#6289=DIRECTION ( 'NONE',  ( 0.000000000000000000, 0.000000000000000000, 1.000000000000000000 ) ) ;
#6292=ORIENTED_EDGE ( 'NONE', *, *, #17759, .F. ) ;
#6293=LINE ( 'NONE', #128, #5099 ) ;
#6298=VECTOR ( 'NONE', #4327, 1000.000000000000000 ) ;
#6316=VECTOR ( 'NONE', #3930, 1000.000000000000000 ) ;
#6323=CARTESIAN_POINT ( 'NONE',  ( -24.79469207716615031, 0.000000000000000000, 1.000000000000000000 ) ) ;
#6325=PLANE ( 'NONE',  #19559 ) ;
#6327=DIRECTION ( 'NONE',  ( 0.000000000000000000, 1.000000000000000000, -0.000000000000000000 ) ) ;
#6331=DIRECTION ( 'NONE',  ( 1.000000000000000000, 0.000000000000000000, 0.000000000000000000 ) ) ;
#6333=DIRECTION ( 'NONE',  ( -0.000000000000000000, -0.000000000000000000, -1.000000000000000000 ) ) ;
#6339=PRODUCT ( 'Moving Upper Ceramic Cutting Blade', 'Moving Upper Ceramic Cutting Blade', '', ( #14733 ) ) ;
#6346=EDGE_LOOP ( 'NONE', ( #12869, #11886, #18495, #1897 ) ) ;
#6348=LINE ( 'NONE', #17431, #5874 ) ;
#6349=ORIENTED_EDGE ( 'NONE', *, *, #17554, .T. ) ;
#6350=CARTESIAN_POINT ( 'NONE',  ( 20.00000000000000000, 5.204170427930421283E-15, 2.000000000000000000 ) ) ;
#6352=DIRECTION ( 'NONE',  ( 0.000000000000000000, 0.000000000000000000, 1.000000000000000000 ) ) ;
#6355=COLOUR_RGB ( '', 0.09019608, 0.27058824, 0.51372549) ;
#6356=VECTOR ( 'NONE', #19393, 1000.000000000000000 ) ;
#6359=DIRECTION ( 'NONE',  ( 0.000000000000000000, 1.000000000000000000, 0.000000000000000000 ) ) ;
#6368=ORIENTED_EDGE ( 'NONE', *, *, #4649, .T. ) ;
#6373=VECTOR ( 'NONE', #1223, 1000.000000000000000 ) ;
#6376=PLANE ( 'NONE',  #7665 ) ;
#6377=VECTOR ( 'NONE', #20046, 1000.000000000000000 ) ;
#6381=ORIENTED_EDGE ( 'NONE', *, *, #13316, .T. ) ;
#6382=EDGE_CURVE ( 'NONE', #16371, #9021, #3617, .T. ) ;
#6386=DIRECTION ( 'NONE',  ( 0.000000000000000000, 0.000000000000000000, 1.000000000000000000 ) ) ;
#6389=VECTOR ( 'NONE', #6230, 1000.000000000000000 ) ;
#6396=PLANE ( 'NONE',  #6731 ) ;
#6410=EDGE_CURVE ( 'NONE', #11562, #15034, #10207, .T. ) ;
#6421=VECTOR ( 'NONE', #7528, 1000.000000000000000 ) ;
#6428=ORIENTED_EDGE ( 'NONE', *, *, #14082, .F. ) ;
#6437=CARTESIAN_POINT ( 'NONE',  ( 0.000000000000000000, 9.000000000000001776, 1.000000000000000000 ) ) ;
#6438=CARTESIAN_POINT ( 'NONE',  ( 20.00000000000000000, 3.500000000000004885, 1.000000000000000000 ) ) ;
#6440=EDGE_CURVE ( 'NONE', #7250, #8074, #2982, .T. ) ;
#6443=CARTESIAN_POINT ( 'NONE',  ( -25.29469207716615031, 9.000000000000001776, 0.000000000000000000 ) ) ;
#6446=CARTESIAN_POINT ( 'NONE',  ( 21.17243175760212637, 9.000000000000001776, 1.000000000000000000 ) ) ;
#6463=CARTESIAN_POINT ( 'NONE',  ( 20.00000000000000000, 3.500000000000004885, 1.500000000000000000 ) ) ;
#6474=LINE ( 'NONE', #8341, #8636 ) ;
#6477=ORIENTED_EDGE ( 'NONE', *, *, #3593, .F. ) ;
#6481=ORIENTED_EDGE ( 'NONE', *, *, #14119, .F. ) ;
#6483=LINE ( 'NONE', #19347, #6995 ) ;
#6487=ADVANCED_FACE ( 'NONE', ( #16254 ), #20662, .T. ) ;
#6489=EDGE_CURVE ( 'NONE', #15669, #15962, #4644, .T. ) ;
#6490=EDGE_LOOP ( 'NONE', ( #16835, #19655, #20339, #5339 ) ) ;
#6493=DIRECTION ( 'NONE',  ( 0.000000000000000000, 0.000000000000000000, 1.000000000000000000 ) ) ;
#6496=PLANE ( 'NONE',  #8359 ) ;
#6511=ORIENTED_EDGE ( 'NONE', *, *, #13005, .T. ) ;
#6512=ORIENTED_EDGE ( 'NONE', *, *, #13469, .T. ) ;
#6515=CARTESIAN_POINT ( 'NONE',  ( 0.000000000000000000, 9.000000000000001776, 1.000000000000000000 ) ) ;
#6527=EDGE_CURVE ( 'NONE', #5550, #3823, #6635, .T. ) ;
#6528=AXIS2_PLACEMENT_3D ( 'NONE', #4963, #9778, #11145 ) ;
#6531=ORIENTED_EDGE ( 'NONE', *, *, #15314, .T. ) ;
#6534=DIRECTION ( 'NONE',  ( 0.000000000000000000, -0.000000000000000000, 1.000000000000000000 ) ) ;
#6536=ORIENTED_EDGE ( 'NONE', *, *, #17673, .T. ) ;
#6539=ORIENTED_EDGE ( 'NONE', *, *, #18899, .T. ) ;
#6544=CARTESIAN_POINT ( 'NONE',  ( 5.999999999999999112, -2.500000000000047518, 2.000000000000000000 ) ) ;
#6546=CARTESIAN_POINT ( 'NONE',  ( 0.000000000000000000, 4.999999999999999112, 0.000000000000000000 ) ) ;
#6552=ORIENTED_EDGE ( 'NONE', *, *, #7078, .F. ) ;
#6554=LINE ( 'NONE', #13331, #22 ) ;
#6556=EDGE_LOOP ( 'NONE', ( #17533, #11540, #11816, #9868 ) ) ;
#6560=EDGE_CURVE ( 'NONE', #17662, #11889, #6219, .T. ) ;
#6561=EDGE_CURVE ( 'NONE', #7456, #20271, #12588, .T. ) ;
#6571=EDGE_CURVE ( 'NONE', #19819, #17249, #3393, .T. ) ;
#6576=ORIENTED_EDGE ( 'NONE', *, *, #11934, .F. ) ;
#6577=VECTOR ( 'NONE', #463, 1000.000000000000000 ) ;
#6579=CARTESIAN_POINT ( 'NONE',  ( 21.17243175760212637, 4.999999999999999112, 0.000000000000000000 ) ) ;
#6580=ORIENTED_EDGE ( 'NONE', *, *, #13085, .T. ) ;
#6584=VECTOR ( 'NONE', #13901, 1000.000000000000000 ) ;
#6585=ORIENTED_EDGE ( 'NONE', *, *, #6561, .T. ) ;
#6586=EDGE_CURVE ( 'NONE', #11965, #15974, #5067, .T. ) ;
#6597=EDGE_CURVE ( 'NONE', #7526, #7096, #13008, .T. ) ;
#6608=ORIENTED_EDGE ( 'NONE', *, *, #2725, .F. ) ;
#6609=DIRECTION ( 'NONE',  ( 1.000000000000000000, 0.000000000000000000, -0.000000000000000000 ) ) ;
#6610=CARTESIAN_POINT ( 'NONE',  ( -22.85856191738413656, 4.999999999999999112, 0.000000000000000000 ) ) ;
#6618=VECTOR ( 'NONE', #2485, 1000.000000000000000 ) ;
#6626=VECTOR ( 'NONE', #18932, 1000.000000000000000 ) ;
#6635=LINE ( 'NONE', #8208, #15094 ) ;
#6636=EDGE_CURVE ( 'NONE', #15034, #9899, #11234, .T. ) ;
#6638=VECTOR ( 'NONE', #3982, 1000.000000000000000 ) ;
#6639=VECTOR ( 'NONE', #15561, 1000.000000000000000 ) ;
#6644=FACE_OUTER_BOUND ( 'NONE', #17413, .T. ) ;
#6645=CYLINDRICAL_SURFACE ( 'NONE', #14306, 0.5000000000000000000 ) ;
#6646=LINE ( 'NONE', #6546, #6718 ) ;
#6648=VECTOR ( 'NONE', #16865, 1000.000000000000000 ) ;
#6649=VERTEX_POINT ( 'NONE', #2329 ) ;
#6658=VECTOR ( 'NONE', #18814, 1000.000000000000114 ) ;
#6660=DIRECTION ( 'NONE',  ( 0.000000000000000000, -0.000000000000000000, 1.000000000000000000 ) ) ;
#6661=ORIENTED_EDGE ( 'NONE', *, *, #12310, .T. ) ;
#6662=DIRECTION ( 'NONE',  ( 0.000000000000000000, -0.000000000000000000, 1.000000000000000000 ) ) ;
#6663=VECTOR ( 'NONE', #10397, 1000.000000000000000 ) ;
#6664=VECTOR ( 'NONE', #10314, 1000.000000000000000 ) ;
#6667=CARTESIAN_POINT ( 'NONE',  ( -17.55017143803810242, 4.999999999999999112, 0.000000000000000000 ) ) ;
#6676=DIRECTION ( 'NONE',  ( 1.000000000000000000, 0.000000000000000000, 0.000000000000000000 ) ) ;
#6678=ORIENTED_EDGE ( 'NONE', *, *, #19139, .F. ) ;
#6682=ORIENTED_EDGE ( 'NONE', *, *, #13605, .F. ) ;
#6684=CARTESIAN_POINT ( 'NONE',  ( 0.000000000000000000, 9.000000000000001776, 1.000000000000000000 ) ) ;
#6691=ORIENTED_EDGE ( 'NONE', *, *, #15226, .T. ) ;
#6698=CYLINDRICAL_SURFACE ( 'NONE', #9682, 0.4999999999999987232 ) ;
#6710=ORIENTED_EDGE ( 'NONE', *, *, #13115, .T. ) ;
#6712=CARTESIAN_POINT ( 'NONE',  ( -23.35856191738413656, 4.999999999999999112, 1.000000000000000000 ) ) ;
#6718=VECTOR ( 'NONE', #11454, 1000.000000000000000 ) ;
#6720=EDGE_CURVE ( 'NONE', #9631, #11562, #13112, .T. ) ;
#6721=VECTOR ( 'NONE', #5872, 1000.000000000000000 ) ;
#6722=EDGE_CURVE ( 'NONE', #1137, #19645, #6744, .T. ) ;
#6724=DIRECTION ( 'NONE',  ( 0.000000000000000000, -0.000000000000000000, 1.000000000000000000 ) ) ;
#6727=DIRECTION ( 'NONE',  ( 1.000000000000000000, 0.000000000000000000, 0.000000000000000000 ) ) ;
#6731=AXIS2_PLACEMENT_3D ( 'NONE', #14022, #20626, #20431 ) ;
#6733=CARTESIAN_POINT ( 'NONE',  ( 5.683390479346035029, 0.000000000000000000, 1.000000000000000000 ) ) ;
#6734=EDGE_CURVE ( 'NONE', #607, #1583, #8611, .T. ) ;
#6738=ORIENTED_EDGE ( 'NONE', *, *, #17284, .F. ) ;
#6743=ORIENTED_EDGE ( 'NONE', *, *, #12092, .T. ) ;
#6744=LINE ( 'NONE', #6838, #10114 ) ;
#6746=EDGE_CURVE ( 'NONE', #8535, #68, #3903, .T. ) ;
#6747=FACE_OUTER_BOUND ( 'NONE', #12821, .T. ) ;
#6752=DIRECTION ( 'NONE',  ( 0.4999999999999948930, 0.8660254037844415942, -0.000000000000000000 ) ) ;
#6753=DIRECTION ( 'NONE',  ( 0.000000000000000000, -1.000000000000000000, 0.000000000000000000 ) ) ;
#6760=EDGE_CURVE ( 'NONE', #9631, #19648, #7155, .T. ) ;
#6764=CARTESIAN_POINT ( 'NONE',  ( -2.061130159782011972, 0.000000000000000000, 1.000000000000000000 ) ) ;
#6765=ORIENTED_EDGE ( 'NONE', *, *, #9673, .T. ) ;
#6766=ORIENTED_EDGE ( 'NONE', *, *, #6561, .F. ) ;
#6770=DIRECTION ( 'NONE',  ( -1.000000000000000000, 0.000000000000000000, 0.000000000000000000 ) ) ;
#6779=LINE ( 'NONE', #13244, #870 ) ;
#6781=ORIENTED_EDGE ( 'NONE', *, *, #17722, .F. ) ;
#6785=ORIENTED_EDGE ( 'NONE', *, *, #5809, .F. ) ;
#6789=ORIENTED_EDGE ( 'NONE', *, *, #12310, .F. ) ;
#6797=DIRECTION ( 'NONE',  ( 0.000000000000000000, -0.000000000000000000, 1.000000000000000000 ) ) ;
#6804=CARTESIAN_POINT ( 'NONE',  ( -17.05017143803810242, 0.000000000000000000, 1.000000000000000000 ) ) ;
#6805=CARTESIAN_POINT ( 'NONE',  ( 25.54469207716615031, 4.999999999999999112, 0.000000000000000000 ) ) ;
#6813=VERTEX_POINT ( 'NONE', #2129 ) ;
#6816=ADVANCED_FACE ( 'NONE', ( #11746 ), #19921, .F. ) ;
#6817=DIRECTION ( 'NONE',  ( 0.000000000000000000, 0.000000000000000000, -1.000000000000000000 ) ) ;
#6820=LINE ( 'NONE', #3092, #18221 ) ;
#6822=PLANE ( 'NONE',  #13719 ) ;
#6838=CARTESIAN_POINT ( 'NONE',  ( 0.000000000000000000, 9.000000000000001776, 1.000000000000000000 ) ) ;
#6839=CARTESIAN_POINT ( 'NONE',  ( -17.55017143803810242, 9.000000000000001776, 1.000000000000000000 ) ) ;
#6840=DIRECTION ( 'NONE',  ( 8.673617379884033500E-16, -1.000000000000000000, 0.000000000000000000 ) ) ;
#6841=EDGE_CURVE ( 'NONE', #20320, #16909, #11637, .T. ) ;
#6844=DIRECTION ( 'NONE',  ( 1.000000000000000000, 0.000000000000000000, 0.000000000000000000 ) ) ;
#6845=DIRECTION ( 'NONE',  ( 1.000000000000000000, 0.000000000000000000, 0.000000000000000000 ) ) ;
#6853=ADVANCED_FACE ( 'NONE', ( #8512 ), #14881, .T. ) ;
#6855=ORIENTED_EDGE ( 'NONE', *, *, #6841, .T. ) ;
#6859=DIRECTION ( 'NONE',  ( 0.000000000000000000, 0.000000000000000000, 1.000000000000000000 ) ) ;
#6861=VERTEX_POINT ( 'NONE', #15192 ) ;
#6864=DIRECTION ( 'NONE',  ( 0.000000000000000000, -1.000000000000000000, 0.000000000000000000 ) ) ;
#6866=ORIENTED_EDGE ( 'NONE', *, *, #18654, .T. ) ;
#6870=FACE_OUTER_BOUND ( 'NONE', #1511, .T. ) ;
#6881=ORIENTED_EDGE ( 'NONE', *, *, #20226, .T. ) ;
#6884=ORIENTED_EDGE ( 'NONE', *, *, #20030, .F. ) ;
#6889=EDGE_LOOP ( 'NONE', ( #10906, #5114, #6789, #8847, #5812, #2727 ) ) ;
#6908=EDGE_CURVE ( 'NONE', #19548, #16322, #18862, .T. ) ;
#6910=ORIENTED_EDGE ( 'NONE', *, *, #20652, .F. ) ;
#6918=EDGE_CURVE ( 'NONE', #19819, #10249, #10809, .T. ) ;
#6922=CARTESIAN_POINT ( 'NONE',  ( -5.999999999999999112, -7.500000000000047073, 8.999999999999998224 ) ) ;
#6925=EDGE_CURVE ( 'NONE', #431, #1458, #13925, .T. ) ;
#6931=ORIENTED_EDGE ( 'NONE', *, *, #5565, .T. ) ;
#6934=CARTESIAN_POINT ( 'NONE',  ( -5.999999999999999112, -7.500000000000047073, 2.000000000000000000 ) ) ;
#6937=DIRECTION ( 'NONE',  ( -0.000000000000000000, -0.000000000000000000, -1.000000000000000000 ) ) ;
#6943=LINE ( 'NONE', #7056, #19456 ) ;
#6945=DIRECTION ( 'NONE',  ( 0.000000000000000000, 1.000000000000000000, -0.000000000000000000 ) ) ;
#6949=PLANE ( 'NONE',  #20682 ) ;
#6959=VERTEX_POINT ( 'NONE', #10592 ) ;
#6960=EDGE_CURVE ( 'NONE', #15703, #5289, #14032, .T. ) ;
#6961=VERTEX_POINT ( 'NONE', #7358 ) ;
#6962=FACE_OUTER_BOUND ( 'NONE', #18728, .T. ) ;
#6968=ORIENTED_EDGE ( 'NONE', *, *, #11128, .F. ) ;
#6978=VECTOR ( 'NONE', #1624, 1000.000000000000000 ) ;
#6982=DIRECTION ( 'NONE',  ( 1.000000000000000000, -1.734723475976807094E-15, 0.000000000000000000 ) ) ;
#6985=ORIENTED_EDGE ( 'NONE', *, *, #12299, .F. ) ;
#6988=ORIENTED_EDGE ( 'NONE', *, *, #15695, .F. ) ;
#6990=LINE ( 'NONE', #19651, #16671 ) ;
#6994=VERTEX_POINT ( 'NONE', #1182 ) ;
#6995=VECTOR ( 'NONE', #9817, 1000.000000000000000 ) ;
#6997=VECTOR ( 'NONE', #19538, 1000.000000000000000 ) ;
#6998=ORIENTED_EDGE ( 'NONE', *, *, #19303, .F. ) ;
#6999=CARTESIAN_POINT ( 'NONE',  ( 26.04469207716615031, 4.999999999999999112, 1.000000000000000000 ) ) ;
#7005=FACE_OUTER_BOUND ( 'NONE', #6889, .T. ) ;
#7009=AXIS2_PLACEMENT_3D ( 'NONE', #17405, #5838, #7793 ) ;
#7025=LINE ( 'NONE', #19796, #7701 ) ;
#7028=DIRECTION ( 'NONE',  ( -1.000000000000000000, 0.000000000000000000, 0.000000000000000000 ) ) ;
#7031=DIRECTION ( 'NONE',  ( -0.000000000000000000, -0.000000000000000000, -1.000000000000000000 ) ) ;
#7034=DIRECTION ( 'NONE',  ( -0.000000000000000000, -0.000000000000000000, -1.000000000000000000 ) ) ;
#7041=EDGE_LOOP ( 'NONE', ( #13329, #6481, #16595, #14055 ) ) ;
#7045=EDGE_LOOP ( 'NONE', ( #1762, #7354, #1236, #11939 ) ) ;
#7047=ADVANCED_FACE ( 'NONE', ( #18760 ), #12157, .T. ) ;
#7048=VERTEX_POINT ( 'NONE', #2853 ) ;
#7052=EDGE_CURVE ( 'NONE', #3720, #14893, #4210, .T. ) ;
#7056=CARTESIAN_POINT ( 'NONE',  ( 23.60856191738414012, 0.000000000000000000, 0.000000000000000000 ) ) ;
#7057=LINE ( 'NONE', #17833, #10390 ) ;
#7058=CIRCLE ( 'NONE', #1388, 0.4999999999999987232 ) ;
#7064=ORIENTED_EDGE ( 'NONE', *, *, #19019, .F. ) ;
#7073=CARTESIAN_POINT ( 'NONE',  ( 0.000000000000000000, 4.999999999999999112, 1.000000000000000000 ) ) ;
#7075=VERTEX_POINT ( 'NONE', #3259 ) ;
#7077=VECTOR ( 'NONE', #20092, 1000.000000000000000 ) ;
#7078=EDGE_CURVE ( 'NONE', #19625, #20251, #12875, .T. ) ;
#7079=EDGE_CURVE ( 'NONE', #13354, #19089, #6293, .T. ) ;
#7083=DIRECTION ( 'NONE',  ( 0.000000000000000000, 0.000000000000000000, 1.000000000000000000 ) ) ;
#7093=VERTEX_POINT ( 'NONE', #16129 ) ;
#7096=VERTEX_POINT ( 'NONE', #4930 ) ;
#7098=EDGE_CURVE ( 'NONE', #12230, #12873, #19277, .T. ) ;
#7099=DIRECTION ( 'NONE',  ( 0.000000000000000000, 1.000000000000000000, -0.000000000000000000 ) ) ;
#7101=VECTOR ( 'NONE', #4547, 1000.000000000000000 ) ;
#7104=ORIENTED_EDGE ( 'NONE', *, *, #5034, .T. ) ;
#7118=CARTESIAN_POINT ( 'NONE',  ( 1.811130159782011528, 4.999999999999999112, 1.000000000000000000 ) ) ;
#7121=VECTOR ( 'NONE', #9003, 1000.000000000000000 ) ;
#7123=EDGE_CURVE ( 'NONE', #12057, #18833, #3063, .T. ) ;
#7124=DIRECTION ( 'NONE',  ( 0.000000000000000000, -1.000000000000000000, 0.000000000000000000 ) ) ;
#7136=FACE_OUTER_BOUND ( 'NONE', #20465, .T. ) ;
#7141=LINE ( 'NONE', #12624, #13860 ) ;
#7144=FACE_OUTER_BOUND ( 'NONE', #3212, .T. ) ;
#7153=VERTEX_POINT ( 'NONE', #17694 ) ;
#7155=LINE ( 'NONE', #14783, #18803 ) ;
#7160=PLANE ( 'NONE',  #4682 ) ;
#7162=EDGE_CURVE ( 'NONE', #4975, #4594, #1488, .T. ) ;
#7175=ORIENTED_EDGE ( 'NONE', *, *, #3747, .F. ) ;
#7177=CARTESIAN_POINT ( 'NONE',  ( 17.80017143803810242, 0.000000000000000000, 1.000000000000000000 ) ) ;
#7183=VECTOR ( 'NONE', #14262, 1000.000000000000000 ) ;
#7187=ADVANCED_FACE ( 'NONE', ( #9330 ), #9535, .T. ) ;
#7198=EDGE_LOOP ( 'NONE', ( #9744, #18158, #4922, #15804 ) ) ;
#7200=CARTESIAN_POINT ( 'NONE',  ( -9.805650798910056309, 9.000000000000001776, 1.000000000000000000 ) ) ;
#7201=CARTESIAN_POINT ( 'NONE',  ( 0.000000000000000000, 4.999999999999999112, 1.000000000000000000 ) ) ;
#7202=VERTEX_POINT ( 'NONE', #19176 ) ;
#7203=ORIENTED_EDGE ( 'NONE', *, *, #16803, .T. ) ;
#7209=LINE ( 'NONE', #10454, #11697 ) ;
#7222=EDGE_LOOP ( 'NONE', ( #1973, #504, #2555, #3560 ) ) ;
#7225=LINE ( 'NONE', #19989, #12589 ) ;
#7229=FACE_OUTER_BOUND ( 'NONE', #1196, .T. ) ;
#7230=CARTESIAN_POINT ( 'NONE',  ( 9.555650798910054533, 4.999999999999999112, 1.000000000000000000 ) ) ;
#7234=EDGE_CURVE ( 'NONE', #17871, #16350, #9437, .T. ) ;
#7241=EDGE_CURVE ( 'NONE', #19, #9082, #1586, .T. ) ;
#7249=DIRECTION ( 'NONE',  ( 0.000000000000000000, -1.000000000000000000, 0.000000000000000000 ) ) ;
#7250=VERTEX_POINT ( 'NONE', #18213 ) ;
#7251=EDGE_CURVE ( 'NONE', #10835, #17227, #13389, .T. ) ;
#7253=DIRECTION ( 'NONE',  ( -1.000000000000000000, 0.000000000000000000, 0.000000000000000000 ) ) ;
#7254=AXIS2_PLACEMENT_3D ( 'NONE', #15769, #1349, #6058 ) ;
#7259=CARTESIAN_POINT ( 'NONE',  ( -20.92243175760212637, 4.999999999999999112, 1.000000000000000000 ) ) ;
#7260=VECTOR ( 'NONE', #19281, 1000.000000000000114 ) ;
#7261=CARTESIAN_POINT ( 'NONE',  ( -21.42243175760212637, 0.000000000000000000, 1.000000000000000000 ) ) ;
#7265=EDGE_LOOP ( 'NONE', ( #10359, #4771, #4584, #3801 ) ) ;
#7278=ORIENTED_EDGE ( 'NONE', *, *, #18139, .T. ) ;
#7280=ORIENTED_EDGE ( 'NONE', *, *, #661, .F. ) ;
#7281=PLANE ( 'NONE',  #4320 ) ;
#7282=CARTESIAN_POINT ( 'NONE',  ( 8.119520639128047890, 9.000000000000001776, 1.000000000000000000 ) ) ;
#7283=CARTESIAN_POINT ( 'NONE',  ( -17.05017143803810242, 0.000000000000000000, 1.000000000000000000 ) ) ;
#7294=EDGE_LOOP ( 'NONE', ( #435, #14277, #5063, #3086 ) ) ;
#7305=FACE_OUTER_BOUND ( 'NONE', #17999, .T. ) ;
#7306=PLANE ( 'NONE',  #18672 ) ;
#7307=VECTOR ( 'NONE', #848, 1000.000000000000000 ) ;
#7322=AXIS2_PLACEMENT_3D ( 'NONE', #8419, #2229, #8614 ) ;
#7325=AXIS2_PLACEMENT_3D ( 'NONE', #1051, #7743, #9409 ) ;
#7327=EDGE_LOOP ( 'NONE', ( #9205, #5739, #9968, #6931 ) ) ;
#7329=CARTESIAN_POINT ( 'NONE',  ( -20.00000000000000000, 2.499999999999999556, 2.000000000000000000 ) ) ;
#7330=VERTEX_POINT ( 'NONE', #16328 ) ;
#7331=EDGE_CURVE ( 'NONE', #20224, #5681, #8586, .T. ) ;
#7332=DIRECTION ( 'NONE',  ( -1.000000000000000000, 0.000000000000000000, 0.000000000000000000 ) ) ;
#7337=VECTOR ( 'NONE', #18895, 1000.000000000000000 ) ;
#7346=EDGE_CURVE ( 'NONE', #15234, #3417, #9845, .T. ) ;
#7347=CARTESIAN_POINT ( 'NONE',  ( 0.000000000000000000, 4.999999999999999112, 1.000000000000000000 ) ) ;
#7351=ORIENTED_EDGE ( 'NONE', *, *, #6720, .T. ) ;
#7354=ORIENTED_EDGE ( 'NONE', *, *, #20628, .F. ) ;
#7355=EDGE_CURVE ( 'NONE', #5494, #1315, #3671, .T. ) ;
#7358=CARTESIAN_POINT ( 'NONE',  ( -3.999999999999999112, -7.500000000000047073, 7.000000000000000000 ) ) ;
#7360=VECTOR ( 'NONE', #13572, 1000.000000000000000 ) ;
#7374=VECTOR ( 'NONE', #17319, 1000.000000000000000 ) ;
#7375=CARTESIAN_POINT ( 'NONE',  ( -2.061130159782011972, 4.999999999999999112, 0.000000000000000000 ) ) ;
#7384=CARTESIAN_POINT ( 'NONE',  ( 4.999999999999998224, -7.500000000000047073, 9.999999999999998224 ) ) ;
#7385=EDGE_CURVE ( 'NONE', #16591, #14054, #8692, .T. ) ;
#7393=AXIS2_PLACEMENT_3D ( 'NONE', #6733, #13100, #11533 ) ;
#7398=EDGE_CURVE ( 'NONE', #15234, #6239, #15063, .T. ) ;
#7412=LINE ( 'NONE', #7200, #10289 ) ;
#7413=PLANE ( 'NONE',  #13666 ) ;
#7418=CARTESIAN_POINT ( 'NONE',  ( -9.305650798910056309, 4.999999999999999112, 1.000000000000000000 ) ) ;
#7419=CARTESIAN_POINT ( 'NONE',  ( 0.000000000000000000, 9.000000000000001776, 1.000000000000000000 ) ) ;
#7422=CARTESIAN_POINT ( 'NONE',  ( -0.1250000000000035805, 0.000000000000000000, 0.000000000000000000 ) ) ;
#7427=EDGE_CURVE ( 'NONE', #15500, #13273, #11517, .T. ) ;
#7434=ORIENTED_EDGE ( 'NONE', *, *, #6960, .F. ) ;
#7437=DIRECTION ( 'NONE',  ( -0.000000000000000000, 0.000000000000000000, -1.000000000000000000 ) ) ;
#7446=CARTESIAN_POINT ( 'NONE',  ( 0.000000000000000000, 9.000000000000001776, 0.000000000000000000 ) ) ;
#7448=PLANE ( 'NONE',  #3073 ) ;
#7450=AXIS2_PLACEMENT_3D ( 'NONE', #559, #6937, #7253 ) ;
#7456=VERTEX_POINT ( 'NONE', #5344 ) ;
#7457=EDGE_CURVE ( 'NONE', #16862, #4975, #10156, .T. ) ;
#7464=VECTOR ( 'NONE', #15884, 1000.000000000000000 ) ;
#7476=VERTEX_POINT ( 'NONE', #15478 ) ;
#7483=DIRECTION ( 'NONE',  ( -0.000000000000000000, 0.000000000000000000, -1.000000000000000000 ) ) ;
#7484=ORIENTED_EDGE ( 'NONE', *, *, #15015, .T. ) ;
#7485=ORIENTED_EDGE ( 'NONE', *, *, #7649, .F. ) ;
#7486=CARTESIAN_POINT ( 'NONE',  ( -20.00000000000000000, 0.000000000000000000, 1.000000000000000000 ) ) ;
#7495=DIRECTION ( 'NONE',  ( 0.000000000000000000, -1.000000000000000000, 0.000000000000000000 ) ) ;
#7499=ADVANCED_FACE ( 'NONE', ( #1058 ), #2831, .F. ) ;
#7502=EDGE_CURVE ( 'NONE', #6961, #16070, #18734, .T. ) ;
#7512=DIRECTION ( 'NONE',  ( 1.000000000000000000, 0.000000000000000000, -0.000000000000000000 ) ) ;
#7513=ORIENTED_EDGE ( 'NONE', *, *, #11530, .F. ) ;
#7515=EDGE_CURVE ( 'NONE', #19129, #5007, #16738, .T. ) ;
#7517=LINE ( 'NONE', #12419, #13310 ) ;
#7518=CARTESIAN_POINT ( 'NONE',  ( 26.04469207716615031, 9.000000000000001776, 0.000000000000000000 ) ) ;
#7522=FACE_OUTER_BOUND ( 'NONE', #12224, .T. ) ;
#7526=VERTEX_POINT ( 'NONE', #16841 ) ;
#7528=DIRECTION ( 'NONE',  ( 0.000000000000000000, -1.000000000000000000, 0.000000000000000000 ) ) ;
#7532=ORIENTED_EDGE ( 'NONE', *, *, #16136, .T. ) ;
#7533=ORIENTED_EDGE ( 'NONE', *, *, #14609, .T. ) ;
#7536=CARTESIAN_POINT ( 'NONE',  ( -9.305650798910056309, 0.000000000000000000, 1.000000000000000000 ) ) ;
#7537=VECTOR ( 'NONE', #9234, 1000.000000000000000 ) ;
#7539=ORIENTED_EDGE ( 'NONE', *, *, #11297, .T. ) ;
#7541=CARTESIAN_POINT ( 'NONE',  ( -3.999999999999999112, -7.500000000000047073, 9.999999999999998224 ) ) ;
#7544=CARTESIAN_POINT ( 'NONE',  ( 0.000000000000000000, 9.000000000000001776, 1.000000000000000000 ) ) ;
#7546=LINE ( 'NONE', #13598, #10391 ) ;
#7549=DIRECTION ( 'NONE',  ( 1.000000000000000000, 0.000000000000000000, -0.000000000000000000 ) ) ;
#7551=CARTESIAN_POINT ( 'NONE',  ( 19.73630159782011617, 0.000000000000000000, 1.000000000000000000 ) ) ;
#7555=EDGE_LOOP ( 'NONE', ( #1774, #19987, #1531, #14561 ) ) ;
#7557=FACE_OUTER_BOUND ( 'NONE', #4275, .T. ) ;
#7565=EDGE_CURVE ( 'NONE', #11462, #7606, #13692, .T. ) ;
#7566=CARTESIAN_POINT ( 'NONE',  ( 17.80017143803810242, 4.999999999999999112, 1.000000000000000000 ) ) ;
#7567=FACE_OUTER_BOUND ( 'NONE', #8998, .T. ) ;
#7574=ORIENTED_EDGE ( 'NONE', *, *, #6039, .F. ) ;
#7579=ORIENTED_EDGE ( 'NONE', *, *, #11635, .F. ) ;
#7595=CARTESIAN_POINT ( 'NONE',  ( 0.000000000000000000, 9.000000000000001776, 0.000000000000000000 ) ) ;
#7598=PLANE ( 'NONE',  #3696 ) ;
#7606=VERTEX_POINT ( 'NONE', #19993 ) ;
#7611=EDGE_CURVE ( 'NONE', #16180, #20415, #16939, .T. ) ;
#7613=FACE_OUTER_BOUND ( 'NONE', #101, .T. ) ;
#7614=CARTESIAN_POINT ( 'NONE',  ( -1.561130159782011306, 9.000000000000001776, 1.000000000000000000 ) ) ;
#7617=LINE ( 'NONE', #15767, #16972 ) ;
#7624=ORIENTED_EDGE ( 'NONE', *, *, #6218, .F. ) ;
#7630=EDGE_LOOP ( 'NONE', ( #10731, #10931, #11082, #385 ) ) ;
#7634=CARTESIAN_POINT ( 'NONE',  ( -17.11324865405191176, -11.00000000000000000, 1.000000000000000000 ) ) ;
#7635=ORIENTED_EDGE ( 'NONE', *, *, #15537, .T. ) ;
#7636=VECTOR ( 'NONE', #19749, 1000.000000000000000 ) ;
#7638=VECTOR ( 'NONE', #9924, 1000.000000000000000 ) ;
#7639=VERTEX_POINT ( 'NONE', #2508 ) ;
#7641=CARTESIAN_POINT ( 'NONE',  ( -17.05017143803810242, 9.000000000000001776, 1.000000000000000000 ) ) ;
#7642=DIRECTION ( 'NONE',  ( -1.000000000000000000, 0.000000000000000000, 0.000000000000000000 ) ) ;
#7646=AXIS2_PLACEMENT_3D ( 'NONE', #3702, #11446, #5069 ) ;
#7649=EDGE_CURVE ( 'NONE', #19969, #18281, #12339, .T. ) ;
#7651=LINE ( 'NONE', #9320, #7730 ) ;
#7659=ORIENTED_EDGE ( 'NONE', *, *, #3263, .T. ) ;
#7664=CARTESIAN_POINT ( 'NONE',  ( -20.00000000000000000, -0.5000000000000004441, 0.5000000000000000000 ) ) ;
#7665=AXIS2_PLACEMENT_3D ( 'NONE', #5111, #98, #9917 ) ;
#7668=CARTESIAN_POINT ( 'NONE',  ( 23.10856191738414012, 4.999999999999999112, 0.000000000000000000 ) ) ;
#7674=ORIENTED_EDGE ( 'NONE', *, *, #7398, .T. ) ;
#7675=VECTOR ( 'NONE', #13643, 1000.000000000000000 ) ;
#7682=EDGE_LOOP ( 'NONE', ( #11972, #16575, #3087, #10720 ) ) ;
#7684=DIRECTION ( 'NONE',  ( 0.000000000000000000, -0.000000000000000000, 1.000000000000000000 ) ) ;
#7686=ORIENTED_EDGE ( 'NONE', *, *, #9232, .T. ) ;
#7689=ORIENTED_EDGE ( 'NONE', *, *, #3638, .F. ) ;
#7691=EDGE_CURVE ( 'NONE', #20689, #12892, #20303, .T. ) ;
#7694=CARTESIAN_POINT ( 'NONE',  ( 19.23630159782011617, 0.000000000000000000, 0.000000000000000000 ) ) ;
#7695=CARTESIAN_POINT ( 'NONE',  ( 7.619520639128047002, 9.000000000000001776, 1.000000000000000000 ) ) ;
#7699=CARTESIAN_POINT ( 'NONE',  ( 24.50000000000000000, 0.000000000000000000, 1.000000000000000000 ) ) ;
#7700=FACE_OUTER_BOUND ( 'NONE', #14085, .T. ) ;
#7701=VECTOR ( 'NONE', #16624, 1000.000000000000000 ) ;
#7715=ORIENTED_EDGE ( 'NONE', *, *, #9847, .F. ) ;
#7718=AXIS2_PLACEMENT_3D ( 'NONE', #7551, #8814, #2629 ) ;
#7725=CARTESIAN_POINT ( 'NONE',  ( 2.311130159782011972, 0.000000000000000000, 1.000000000000000000 ) ) ;
#7727=CARTESIAN_POINT ( 'NONE',  ( 15.86404127825609400, 0.000000000000000000, 1.000000000000000000 ) ) ;
#7730=VECTOR ( 'NONE', #12551, 1000.000000000000000 ) ;
#7732=SURFACE_SIDE_STYLE ('',( #2915 ) ) ;
#7734=VECTOR ( 'NONE', #10266, 1000.000000000000000 ) ;
#7736=VERTEX_POINT ( 'NONE', #19251 ) ;
#7738=CARTESIAN_POINT ( 'NONE',  ( 9.555650798910054533, 9.000000000000001776, 1.000000000000000000 ) ) ;
#7743=DIRECTION ( 'NONE',  ( 1.000000000000000000, 0.000000000000000000, -0.000000000000000000 ) ) ;
#7752=DIRECTION ( 'NONE',  ( 1.000000000000000000, 0.000000000000000000, 0.000000000000000000 ) ) ;
#7762=VECTOR ( 'NONE', #11037, 1000.000000000000000 ) ;
#7765=ORIENTED_EDGE ( 'NONE', *, *, #17591, .F. ) ;
#7768=ORIENTED_EDGE ( 'NONE', *, *, #14481, .T. ) ;
#7769=UNCERTAINTY_MEASURE_WITH_UNIT (LENGTH_MEASURE( 1.000000000000000082E-05 ), #18732, 'distance_accuracy_value', 'NONE');
#7770=VECTOR ( 'NONE', #230, 1000.000000000000000 ) ;
#7773=EDGE_CURVE ( 'NONE', #4874, #17458, #11090, .T. ) ;
#7778=LINE ( 'NONE', #20642, #4709 ) ;
#7779=LINE ( 'NONE', #13930, #10884 ) ;
#7780=DIRECTION ( 'NONE',  ( 1.000000000000000000, 0.000000000000000000, 0.000000000000000000 ) ) ;
#7793=DIRECTION ( 'NONE',  ( -0.000000000000000000, 0.000000000000000000, -1.000000000000000000 ) ) ;
#7795=VECTOR ( 'NONE', #20102, 1000.000000000000000 ) ;
#7798=EDGE_CURVE ( 'NONE', #8356, #15336, #9308, .T. ) ;
#7814=ORIENTED_EDGE ( 'NONE', *, *, #11983, .T. ) ;
#7817=ORIENTED_EDGE ( 'NONE', *, *, #9887, .F. ) ;
#7835=CARTESIAN_POINT ( 'NONE',  ( 11.99178095869207006, 9.000000000000001776, 1.000000000000000000 ) ) ;
#7845=ORIENTED_EDGE ( 'NONE', *, *, #16549, .F. ) ;
#7847=CARTESIAN_POINT ( 'NONE',  ( -22.85856191738413656, 0.000000000000000000, 1.000000000000000000 ) ) ;
#7857=VECTOR ( 'NONE', #3985, 1000.000000000000000 ) ;
#7858=EDGE_CURVE ( 'NONE', #4979, #7476, #1773, .T. ) ;
#7861=ORIENTED_EDGE ( 'NONE', *, *, #5885, .T. ) ;
#7863=PLANE ( 'NONE',  #12003 ) ;
#7864=ORIENTED_EDGE ( 'NONE', *, *, #14858, .F. ) ;
#7865=ORIENTED_EDGE ( 'NONE', *, *, #3709, .F. ) ;
#7868=ADVANCED_FACE ( 'NONE', ( #6267 ), #18838, .F. ) ;
#7875=CARTESIAN_POINT ( 'NONE',  ( 0.000000000000000000, 4.999999999999999112, 1.000000000000000000 ) ) ;
#7884=EDGE_CURVE ( 'NONE', #17458, #12251, #3037, .T. ) ;
#7889=DIRECTION ( 'NONE',  ( 0.000000000000000000, 1.000000000000000000, -0.000000000000000000 ) ) ;
#7897=LINE ( 'NONE', #18993, #2001 ) ;
#7900=CARTESIAN_POINT ( 'NONE',  ( -7.369520639128046113, 9.000000000000001776, 1.000000000000000000 ) ) ;
#7902=CARTESIAN_POINT ( 'NONE',  ( 4.247260319564023945, 0.000000000000000000, 1.000000000000000000 ) ) ;
#7903=CARTESIAN_POINT ( 'NONE',  ( 3.747260319564023501, 4.999999999999999112, 1.000000000000000000 ) ) ;
#7916=VERTEX_POINT ( 'NONE', #19654 ) ;
#7917=CARTESIAN_POINT ( 'NONE',  ( 0.000000000000000000, 4.999999999999999112, 1.000000000000000000 ) ) ;
#7920=PLANE ( 'NONE',  #2953 ) ;
#7922=CARTESIAN_POINT ( 'NONE',  ( 0.000000000000000000, 4.999999999999999112, 1.000000000000000000 ) ) ;
#7931=ORIENTED_EDGE ( 'NONE', *, *, #16394, .T. ) ;
#7934=DIRECTION ( 'NONE',  ( -0.000000000000000000, -0.000000000000000000, -1.000000000000000000 ) ) ;
#7936=LINE ( 'NONE', #12537, #14263 ) ;
#7940=ORIENTED_EDGE ( 'NONE', *, *, #16763, .F. ) ;
#7943=DIRECTION ( 'NONE',  ( 1.000000000000000000, 0.000000000000000000, 0.000000000000000000 ) ) ;
#7949=LINE ( 'NONE', #3353, #2034 ) ;
#7970=VECTOR ( 'NONE', #11148, 1000.000000000000000 ) ;
#7983=ORIENTED_EDGE ( 'NONE', *, *, #9887, .T. ) ;
#7988=VECTOR ( 'NONE', #17511, 1000.000000000000000 ) ;
#7989=FACE_OUTER_BOUND ( 'NONE', #19918, .T. ) ;
#7990=ORIENTED_EDGE ( 'NONE', *, *, #15577, .T. ) ;
#7992=EDGE_LOOP ( 'NONE', ( #19405, #2545, #1114, #6710 ) ) ;
#7993=DIRECTION ( 'NONE',  ( -0.000000000000000000, -0.000000000000000000, -1.000000000000000000 ) ) ;
#8001=CARTESIAN_POINT ( 'NONE',  ( 0.000000000000000000, 9.000000000000001776, 0.000000000000000000 ) ) ;
#8005=FACE_OUTER_BOUND ( 'NONE', #9863, .T. ) ;
#8011=AXIS2_PLACEMENT_3D ( 'NONE', #4171, #2596, #8784 ) ;
#8017=CARTESIAN_POINT ( 'NONE',  ( -9.805650798910056309, 4.999999999999999112, 1.000000000000000000 ) ) ;
#8019=VERTEX_POINT ( 'NONE', #12285 ) ;
#8022=ORIENTED_EDGE ( 'NONE', *, *, #6560, .F. ) ;
#8024=AXIS2_PLACEMENT_3D ( 'NONE', #4834, #3265, #8086 ) ;
#8026=ORIENTED_EDGE ( 'NONE', *, *, #10465, .T. ) ;
#8029=EDGE_CURVE ( 'NONE', #14610, #381, #18613, .T. ) ;
#8030=DIRECTION ( 'NONE',  ( 1.000000000000000000, 0.000000000000000000, -0.000000000000000000 ) ) ;
#8045=VECTOR ( 'NONE', #15588, 1000.000000000000000 ) ;
#8048=VECTOR ( 'NONE', #15330, 1000.000000000000000 ) ;
#8051=ORIENTED_EDGE ( 'NONE', *, *, #4274, .T. ) ;
#8054=ORIENTED_EDGE ( 'NONE', *, *, #4678, .F. ) ;
#8060=PLANE ( 'NONE',  #14811 ) ;
#8065=CARTESIAN_POINT ( 'NONE',  ( 0.000000000000000000, 4.999999999999999112, 0.000000000000000000 ) ) ;
#8074=VERTEX_POINT ( 'NONE', #12590 ) ;
#8075=ORIENTED_EDGE ( 'NONE', *, *, #20385, .T. ) ;
#8077=DIRECTION ( 'NONE',  ( -0.000000000000000000, -0.000000000000000000, -1.000000000000000000 ) ) ;
#8078=LINE ( 'NONE', #8384, #1341 ) ;
#8083=CARTESIAN_POINT ( 'NONE',  ( 17.11324865405191176, -10.99999999999999645, 2.000000000000000000 ) ) ;
#8086=DIRECTION ( 'NONE',  ( 0.000000000000000000, -0.000000000000000000, 1.000000000000000000 ) ) ;
#8091=DIRECTION ( 'NONE',  ( -1.000000000000000000, 0.000000000000000000, 0.000000000000000000 ) ) ;
#8093=VECTOR ( 'NONE', #9708, 1000.000000000000000 ) ;
#8105=DIRECTION ( 'NONE',  ( 0.000000000000000000, -0.000000000000000000, 1.000000000000000000 ) ) ;
#8107=EDGE_LOOP ( 'NONE', ( #12768, #20207, #16906, #6071 ) ) ;
#8111=EDGE_CURVE ( 'NONE', #8663, #16909, #3514, .T. ) ;
#8117=CARTESIAN_POINT ( 'NONE',  ( -13.67791111847408025, 0.000000000000000000, 1.000000000000000000 ) ) ;
#8125=ORIENTED_EDGE ( 'NONE', *, *, #17284, .T. ) ;
#8127=CARTESIAN_POINT ( 'NONE',  ( -20.00000000000000000, 2.499999999999999556, 1.500000000000000000 ) ) ;
#8128=ORIENTED_EDGE ( 'NONE', *, *, #7346, .T. ) ;
#8129=EDGE_CURVE ( 'NONE', #13158, #13679, #10618, .T. ) ;
#8130=ORIENTED_EDGE ( 'NONE', *, *, #10257, .F. ) ;
#8131=FACE_OUTER_BOUND ( 'NONE', #13954, .T. ) ;
#8134=AXIS2_PLACEMENT_3D ( 'NONE', #14839, #16602, #16824 ) ;
#8136=LINE ( 'NONE', #17439, #17337 ) ;
#8139=EDGE_CURVE ( 'NONE', #12892, #12897, #11445, .T. ) ;
#8140=ADVANCED_FACE ( 'NONE', ( #5164 ), #11544, .T. ) ;
#8146=CARTESIAN_POINT ( 'NONE',  ( 27.49999999999999645, -4.770489558936219510E-14, 1.000000000000000000 ) ) ;
#8153=ORIENTED_EDGE ( 'NONE', *, *, #1822, .F. ) ;
#8154=EDGE_CURVE ( 'NONE', #12948, #2020, #16051, .T. ) ;
#8156=PLANE ( 'NONE',  #12331 ) ;
#8157=VERTEX_POINT ( 'NONE', #360 ) ;
#8159=CARTESIAN_POINT ( 'NONE',  ( 0.000000000000000000, 9.000000000000001776, 1.000000000000000000 ) ) ;
#8161=ORIENTED_EDGE ( 'NONE', *, *, #14609, .F. ) ;
#8164=FACE_OUTER_BOUND ( 'NONE', #15785, .T. ) ;
#8176=ORIENTED_EDGE ( 'NONE', *, *, #20498, .F. ) ;
#8180=DIRECTION ( 'NONE',  ( 1.000000000000000000, 0.000000000000000000, 0.000000000000000000 ) ) ;
#8183=CARTESIAN_POINT ( 'NONE',  ( -18.98630159782011262, 0.000000000000000000, 1.000000000000000000 ) ) ;
#8184=CARTESIAN_POINT ( 'NONE',  ( 0.000000000000000000, 0.000000000000000000, 2.000000000000000000 ) ) ;
#8188=CARTESIAN_POINT ( 'NONE',  ( 0.000000000000000000, 0.000000000000000000, 1.000000000000000000 ) ) ;
#8192=LINE ( 'NONE', #1496, #5399 ) ;
#8197=LINE ( 'NONE', #12995, #2712 ) ;
#8201=ORIENTED_EDGE ( 'NONE', *, *, #4382, .F. ) ;
#8204=CARTESIAN_POINT ( 'NONE',  ( 3.999999999999999112, -2.500000000000047518, 9.999999999999998224 ) ) ;
#8207=ORIENTED_EDGE ( 'NONE', *, *, #7052, .F. ) ;
#8208=CARTESIAN_POINT ( 'NONE',  ( 17.80017143803810242, 9.000000000000001776, 1.000000000000000000 ) ) ;
#8209=DIRECTION ( 'NONE',  ( 1.000000000000000000, 0.000000000000000000, 0.000000000000000000 ) ) ;
#8212=EDGE_LOOP ( 'NONE', ( #14420, #16231, #13565, #9154 ) ) ;
#8218=DIRECTION ( 'NONE',  ( 0.000000000000000000, -1.000000000000000000, 0.000000000000000000 ) ) ;
#8227=LINE ( 'NONE', #13027, #2697 ) ;
#8229=ORIENTED_EDGE ( 'NONE', *, *, #19634, .T. ) ;
#8230=CARTESIAN_POINT ( 'NONE',  ( 20.00000000000000000, -5.999999999999994671, 1.000000000000000000 ) ) ;
#8233=DIRECTION ( 'NONE',  ( 0.000000000000000000, 1.000000000000000000, -0.000000000000000000 ) ) ;
#8234=VECTOR ( 'NONE', #942, 1000.000000000000000 ) ;
#8235=ORIENTED_EDGE ( 'NONE', *, *, #1510, .T. ) ;
#8239=DIRECTION ( 'NONE',  ( -0.000000000000000000, 0.000000000000000000, -1.000000000000000000 ) ) ;
#8244=VERTEX_POINT ( 'NONE', #17507 ) ;
#8251=ADVANCED_FACE ( 'NONE', ( #3189 ), #14681, .T. ) ;
#8254=ORIENTED_EDGE ( 'NONE', *, *, #15314, .F. ) ;
#8258=ORIENTED_EDGE ( 'NONE', *, *, #18205, .F. ) ;
#8263=CARTESIAN_POINT ( 'NONE',  ( -7.369520639128046113, 4.999999999999999112, 1.000000000000000000 ) ) ;
#8274=ORIENTED_EDGE ( 'NONE', *, *, #4716, .T. ) ;
#8276=CARTESIAN_POINT ( 'NONE',  ( -9.305650798910056309, 4.999999999999999112, 0.000000000000000000 ) ) ;
#8277=ORIENTED_EDGE ( 'NONE', *, *, #10161, .T. ) ;
#8281=VECTOR ( 'NONE', #12306, 1000.000000000000000 ) ;
#8285=CARTESIAN_POINT ( 'NONE',  ( -23.35856191738413656, 4.999999999999999112, 1.000000000000000000 ) ) ;
#8294=PLANE ( 'NONE',  #7393 ) ;
#8303=DIRECTION ( 'NONE',  ( -0.000000000000000000, -0.000000000000000000, -1.000000000000000000 ) ) ;
#8314=LINE ( 'NONE', #17622, #3302 ) ;
#8315=FACE_OUTER_BOUND ( 'NONE', #15265, .T. ) ;
#8318=ORIENTED_EDGE ( 'NONE', *, *, #19045, .F. ) ;
#8323=ORIENTED_EDGE ( 'NONE', *, *, #11576, .T. ) ;
#8327=ORIENTED_EDGE ( 'NONE', *, *, #19609, .F. ) ;
#8332=VERTEX_POINT ( 'NONE', #4958 ) ;
#8339=VECTOR ( 'NONE', #12513, 1000.000000000000000 ) ;
#8341=CARTESIAN_POINT ( 'NONE',  ( 3.747260319564023501, 0.000000000000000000, 1.000000000000000000 ) ) ;
#8343=LINE ( 'NONE', #13149, #14216 ) ;
#8345=ORIENTED_EDGE ( 'NONE', *, *, #14717, .T. ) ;
#8350=VECTOR ( 'NONE', #14062, 1000.000000000000114 ) ;
#8353=CARTESIAN_POINT ( 'NONE',  ( 19.23630159782011617, 4.999999999999999112, 1.000000000000000000 ) ) ;
#8356=VERTEX_POINT ( 'NONE', #6839 ) ;
#8359=AXIS2_PLACEMENT_3D ( 'NONE', #6180, #4601, #19259 ) ;
#8365=PLANE ( 'NONE',  #15465 ) ;
#8375=VECTOR ( 'NONE', #19994, 1000.000000000000000 ) ;
#8376=LINE ( 'NONE', #13173, #3043 ) ;
#8384=CARTESIAN_POINT ( 'NONE',  ( -7.369520639128046113, 9.000000000000001776, 1.000000000000000000 ) ) ;
#8387=DIRECTION ( 'NONE',  ( -0.000000000000000000, -0.000000000000000000, -1.000000000000000000 ) ) ;
#8388=PLANE ( 'NONE',  #1681 ) ;
#8389=VECTOR ( 'NONE', #12690, 1000.000000000000000 ) ;
#8394=LINE ( 'NONE', #7694, #14526 ) ;
#8396=AXIS2_PLACEMENT_3D ( 'NONE', #10088, #17832, #775 ) ;
#8402=CARTESIAN_POINT ( 'NONE',  ( 19.73630159782011617, 4.999999999999999112, 1.000000000000000000 ) ) ;
#8406=LINE ( 'NONE', #3579, #10060 ) ;
#8413=LINE ( 'NONE', #5160, #16351 ) ;
#8416=ORIENTED_EDGE ( 'NONE', *, *, #5009, .F. ) ;
#8419=CARTESIAN_POINT ( 'NONE',  ( 21.67243175760212637, 0.000000000000000000, 1.000000000000000000 ) ) ;
#8423=CARTESIAN_POINT ( 'NONE',  ( 0.000000000000000000, 9.000000000000001776, 1.000000000000000000 ) ) ;
#8427=LINE ( 'NONE', #19520, #18675 ) ;
#8434=VERTEX_POINT ( 'NONE', #8828 ) ;
#8436=CARTESIAN_POINT ( 'NONE',  ( -20.00000000000000000, 3.000000000000000888, 1.500000000000000000 ) ) ;
#8437=EDGE_LOOP ( 'NONE', ( #9586, #13334, #20512, #17372 ) ) ;
#8439=AXIS2_PLACEMENT_3D ( 'NONE', #11443, #1821, #9666 ) ;
#8447=EDGE_CURVE ( 'NONE', #10249, #16180, #14785, .T. ) ;
#8448=CARTESIAN_POINT ( 'NONE',  ( 0.000000000000000000, 4.999999999999999112, 1.000000000000000000 ) ) ;
#8450=VECTOR ( 'NONE', #1083, 1000.000000000000000 ) ;
#8459=ORIENTED_EDGE ( 'NONE', *, *, #14847, .T. ) ;
#8465=EDGE_CURVE ( 'NONE', #458, #510, #20023, .T. ) ;
#8468=CARTESIAN_POINT ( 'NONE',  ( 25.54469207716615031, 0.000000000000000000, 1.000000000000000000 ) ) ;
#8474=DIRECTION ( 'NONE',  ( -0.1736481776669295263, -0.9848077530122082424, 0.000000000000000000 ) ) ;
#8482=ORIENTED_EDGE ( 'NONE', *, *, #11405, .T. ) ;
#8483=ORIENTED_EDGE ( 'NONE', *, *, #6918, .T. ) ;
#8485=DIRECTION ( 'NONE',  ( 1.000000000000000000, 0.000000000000000000, -0.000000000000000000 ) ) ;
#8488=EDGE_CURVE ( 'NONE', #19095, #5490, #2913, .T. ) ;
#8495=LINE ( 'NONE', #14864, #6050 ) ;
#8498=LINE ( 'NONE', #14965, #14063 ) ;
#8504=ORIENTED_EDGE ( 'NONE', *, *, #545, .T. ) ;
#8507=CARTESIAN_POINT ( 'NONE',  ( -14.00000000000000000, 0.000000000000000000, 2.000000000000000000 ) ) ;
#8508=ORIENTED_EDGE ( 'NONE', *, *, #5199, .T. ) ;
#8510=ORIENTED_EDGE ( 'NONE', *, *, #11576, .F. ) ;
#8512=FACE_OUTER_BOUND ( 'NONE', #8212, .T. ) ;
#8517=LINE ( 'NONE', #9977, #47 ) ;
#8518=CARTESIAN_POINT ( 'NONE',  ( 17.30017143803810242, 0.000000000000000000, 0.000000000000000000 ) ) ;
#8519=EDGE_CURVE ( 'NONE', #3752, #10986, #17266, .T. ) ;
#8520=CARTESIAN_POINT ( 'NONE',  ( 3.747260319564023501, 9.000000000000001776, 1.000000000000000000 ) ) ;
#8524=ORIENTED_EDGE ( 'NONE', *, *, #4414, .T. ) ;
#8528=ORIENTED_EDGE ( 'NONE', *, *, #11089, .F. ) ;
#8530=AXIS2_PLACEMENT_3D ( 'NONE', #10368, #3881, #20107 ) ;
#8531=CARTESIAN_POINT ( 'NONE',  ( -17.55017143803810242, 9.000000000000001776, 1.000000000000000000 ) ) ;
#8533=ORIENTED_EDGE ( 'NONE', *, *, #10567, .T. ) ;
#8535=VERTEX_POINT ( 'NONE', #9029 ) ;
#8540=LINE ( 'NONE', #13142, #14657 ) ;
#8541=CARTESIAN_POINT ( 'NONE',  ( 5.999999999999999112, -7.500000000000047073, 9.999999999999998224 ) ) ;
#8548=CARTESIAN_POINT ( 'NONE',  ( -20.92243175760212637, 0.000000000000000000, 0.000000000000000000 ) ) ;
#8551=ORIENTED_EDGE ( 'NONE', *, *, #11089, .T. ) ;
#8554=ORIENTED_EDGE ( 'NONE', *, *, #16038, .F. ) ;
#8555=PLANE ( 'NONE',  #15959 ) ;
#8556=FACE_OUTER_BOUND ( 'NONE', #9738, .T. ) ;
#8563=DIRECTION ( 'NONE',  ( 0.000000000000000000, -1.000000000000000000, 0.000000000000000000 ) ) ;
#8567=CARTESIAN_POINT ( 'NONE',  ( 5.683390479346035029, 4.999999999999999112, 1.000000000000000000 ) ) ;
#8578=LINE ( 'NONE', #627, #4319 ) ;
#8583=CARTESIAN_POINT ( 'NONE',  ( -19.48630159782011262, 4.999999999999999112, 1.000000000000000000 ) ) ;
#8586=LINE ( 'NONE', #5451, #20150 ) ;
#8587=LINE ( 'NONE', #14955, #1029 ) ;
#8592=CARTESIAN_POINT ( 'NONE',  ( -21.42243175760212637, 4.999999999999999112, 1.000000000000000000 ) ) ;
#8595=CARTESIAN_POINT ( 'NONE',  ( -19.48630159782011262, 9.000000000000001776, 1.000000000000000000 ) ) ;
#8603=ORIENTED_EDGE ( 'NONE', *, *, #14717, .F. ) ;
#8611=LINE ( 'NONE', #11848, #19821 ) ;
#8614=DIRECTION ( 'NONE',  ( -0.000000000000000000, 0.000000000000000000, -1.000000000000000000 ) ) ;
#8617=DIRECTION ( 'NONE',  ( 0.000000000000000000, 1.000000000000000000, -0.000000000000000000 ) ) ;
#8618=DIRECTION ( 'NONE',  ( -0.000000000000000000, -0.000000000000000000, -1.000000000000000000 ) ) ;
#8621=CARTESIAN_POINT ( 'NONE',  ( 0.000000000000000000, 9.000000000000001776, 1.000000000000000000 ) ) ;
#8624=ADVANCED_FACE ( 'NONE', ( #1701 ), #14448, .T. ) ;
#8634=ORIENTED_EDGE ( 'NONE', *, *, #19862, .F. ) ;
#8636=VECTOR ( 'NONE', #9592, 1000.000000000000000 ) ;
#8637=ORIENTED_EDGE ( 'NONE', *, *, #14119, .T. ) ;
#8645=EDGE_CURVE ( 'NONE', #2799, #13818, #19179, .T. ) ;
#8648=CARTESIAN_POINT ( 'NONE',  ( 5.999999999999999112, -7.500000000000047073, 9.999999999999998224 ) ) ;
#8658=CARTESIAN_POINT ( 'NONE',  ( 7.619520639128047002, 0.000000000000000000, 1.000000000000000000 ) ) ;
#8659=DIRECTION ( 'NONE',  ( -0.1736481776669295540, 0.9848077530122082424, 0.000000000000000000 ) ) ;
#8660=ORIENTED_EDGE ( 'NONE', *, *, #13815, .F. ) ;
#8663=VERTEX_POINT ( 'NONE', #5661 ) ;
#8665=AXIS2_PLACEMENT_3D ( 'NONE', #11891, #16703, #3845 ) ;
#8667=ORIENTED_EDGE ( 'NONE', *, *, #8447, .T. ) ;
#8680=VERTEX_POINT ( 'NONE', #15581 ) ;
#8690=DIRECTION ( 'NONE',  ( -0.000000000000000000, -0.000000000000000000, -1.000000000000000000 ) ) ;
#8692=LINE ( 'NONE', #5236, #4111 ) ;
#8694=CARTESIAN_POINT ( 'NONE',  ( 5.683390479346035029, 9.000000000000001776, 0.000000000000000000 ) ) ;
#8718=VERTEX_POINT ( 'NONE', #2834 ) ;
#8721=EDGE_CURVE ( 'NONE', #15336, #20292, #5768, .T. ) ;
#8722=CARTESIAN_POINT ( 'NONE',  ( 11.49178095869207006, 0.000000000000000000, 0.000000000000000000 ) ) ;
#8728=VECTOR ( 'NONE', #20530, 1000.000000000000000 ) ;
#8730=CARTESIAN_POINT ( 'NONE',  ( 5.999999999999999112, -2.500000000000047518, 9.999999999999998224 ) ) ;
#8731=VECTOR ( 'NONE', #3477, 1000.000000000000000 ) ;
#8733=FACE_OUTER_BOUND ( 'NONE', #7041, .T. ) ;
#8743=CARTESIAN_POINT ( 'NONE',  ( -20.00000000000000000, 0.000000000000000000, 2.000000000000000000 ) ) ;
#8745=VERTEX_POINT ( 'NONE', #12238 ) ;
#8749=VECTOR ( 'NONE', #16715, 1000.000000000000000 ) ;
#8751=ORIENTED_EDGE ( 'NONE', *, *, #2628, .F. ) ;
#8754=CARTESIAN_POINT ( 'NONE',  ( 0.000000000000000000, 9.000000000000001776, 0.000000000000000000 ) ) ;
#8758=CARTESIAN_POINT ( 'NONE',  ( -15.11404127825609223, 4.999999999999999112, 1.000000000000000000 ) ) ;
#8765=ORIENTED_EDGE ( 'NONE', *, *, #5646, .F. ) ;
#8768=ORIENTED_EDGE ( 'NONE', *, *, #19901, .F. ) ;
#8770=CARTESIAN_POINT ( 'NONE',  ( -22.85856191738413656, 0.000000000000000000, 1.000000000000000000 ) ) ;
#8771=EDGE_LOOP ( 'NONE', ( #18467, #6191, #5176, #8637 ) ) ;
#8772=ORIENTED_EDGE ( 'NONE', *, *, #13316, .F. ) ;
#8773=ADVANCED_FACE ( 'NONE', ( #20306 ), #12448, .T. ) ;
#8774=ADVANCED_FACE ( 'NONE', ( #4505 ), #5968, .T. ) ;
#8775=EDGE_LOOP ( 'NONE', ( #15369, #791, #17864, #1580 ) ) ;
#8776=DIRECTION ( 'NONE',  ( 0.000000000000000000, 0.000000000000000000, -1.000000000000000000 ) ) ;
#8778=CARTESIAN_POINT ( 'NONE',  ( -26.04469207716614676, 4.999999999999999112, 0.000000000000000000 ) ) ;
#8779=ADVANCED_FACE ( 'NONE', ( #12343 ), #18737, .T. ) ;
#8781=CARTESIAN_POINT ( 'NONE',  ( 0.000000000000000000, 4.999999999999999112, 1.000000000000000000 ) ) ;
#8783=CYLINDRICAL_SURFACE ( 'NONE', #18439, 2.999999999999999112 ) ;
#8784=DIRECTION ( 'NONE',  ( 0.000000000000000000, 0.000000000000000000, 1.000000000000000000 ) ) ;
#8797=ORIENTED_EDGE ( 'NONE', *, *, #6286, .F. ) ;
#8799=LINE ( 'NONE', #8898, #548 ) ;
#8804=LINE ( 'NONE', #18118, #1957 ) ;
#8806=CARTESIAN_POINT ( 'NONE',  ( -2.061130159782011972, 9.000000000000001776, 1.000000000000000000 ) ) ;
#8810=CARTESIAN_POINT ( 'NONE',  ( 0.000000000000000000, 4.999999999999999112, 0.000000000000000000 ) ) ;
#8814=DIRECTION ( 'NONE',  ( 1.000000000000000000, 0.000000000000000000, -0.000000000000000000 ) ) ;
#8827=VECTOR ( 'NONE', #6027, 1000.000000000000000 ) ;
#8828=CARTESIAN_POINT ( 'NONE',  ( 13.42791111847407848, 9.000000000000001776, 0.000000000000000000 ) ) ;
#8832=DIRECTION ( 'NONE',  ( -0.000000000000000000, -0.000000000000000000, -1.000000000000000000 ) ) ;
#8845=DIRECTION ( 'NONE',  ( -1.000000000000000000, 0.000000000000000000, 0.000000000000000000 ) ) ;
#8847=ORIENTED_EDGE ( 'NONE', *, *, #8029, .T. ) ;
#8849=ORIENTED_EDGE ( 'NONE', *, *, #1690, .T. ) ;
#8853=DIRECTION ( 'NONE',  ( 0.000000000000000000, 1.000000000000000000, 0.000000000000000000 ) ) ;
#8855=CARTESIAN_POINT ( 'NONE',  ( 13.92791111847407848, 9.000000000000001776, 1.000000000000000000 ) ) ;
#8858=VECTOR ( 'NONE', #2812, 1000.000000000000000 ) ;
#8869=ORIENTED_EDGE ( 'NONE', *, *, #4630, .T. ) ;
#8871=CARTESIAN_POINT ( 'NONE',  ( 13.50000000000000178, 7.806255641895631925E-15, 2.000000000000000000 ) ) ;
#8872=ORIENTED_EDGE ( 'NONE', *, *, #17986, .T. ) ;
#8876=EDGE_CURVE ( 'NONE', #20251, #3865, #12643, .T. ) ;
#8877=CARTESIAN_POINT ( 'NONE',  ( 0.000000000000000000, 4.999999999999999112, 1.000000000000000000 ) ) ;
#8882=LINE ( 'NONE', #1037, #337 ) ;
#8886=EDGE_CURVE ( 'NONE', #3209, #15372, #12953, .T. ) ;
#8887=ORIENTED_EDGE ( 'NONE', *, *, #4755, .T. ) ;
#8888=ADVANCED_FACE ( 'NONE', ( #5013 ), #12853, .T. ) ;
#8894=PLANE ( 'NONE',  #18008 ) ;
#8898=CARTESIAN_POINT ( 'NONE',  ( -9.305650798910056309, 0.000000000000000000, 0.000000000000000000 ) ) ;
#8901=LINE ( 'NONE', #3878, #8375 ) ;
#8912=CARTESIAN_POINT ( 'NONE',  ( -13.50000000000000178, 0.000000000000000000, 1.000000000000000000 ) ) ;
#8922=EDGE_CURVE ( 'NONE', #17043, #11975, #14933, .T. ) ;
#8926=DIRECTION ( 'NONE',  ( -0.000000000000000000, -0.000000000000000000, -1.000000000000000000 ) ) ;
#8929=CARTESIAN_POINT ( 'NONE',  ( -3.997260319564023501, 0.000000000000000000, 0.000000000000000000 ) ) ;
#8938=ORIENTED_EDGE ( 'NONE', *, *, #2318, .F. ) ;
#8940=DIRECTION ( 'NONE',  ( 0.000000000000000000, -1.000000000000000000, 0.000000000000000000 ) ) ;
#8947=DIRECTION ( 'NONE',  ( -0.000000000000000000, 0.000000000000000000, -1.000000000000000000 ) ) ;
#8949=EDGE_CURVE ( 'NONE', #11770, #1149, #11595, .T. ) ;
#8950=CARTESIAN_POINT ( 'NONE',  ( 0.000000000000000000, 9.000000000000001776, 0.000000000000000000 ) ) ;
#8952=LINE ( 'NONE', #10738, #3846 ) ;
#8954=PLANE ( 'NONE',  #9307 ) ;
#8955=CARTESIAN_POINT ( 'NONE',  ( 13.42791111847407848, 4.999999999999999112, 1.000000000000000000 ) ) ;
#8958=DIRECTION ( 'NONE',  ( 1.734723475976807094E-15, 1.000000000000000000, 0.000000000000000000 ) ) ;
#8961=VECTOR ( 'NONE', #17760, 1000.000000000000000 ) ;
#8962=ORIENTED_EDGE ( 'NONE', *, *, #4983, .T. ) ;
#8966=VECTOR ( 'NONE', #18510, 1000.000000000000000 ) ;
#8967=PLANE ( 'NONE',  #5270 ) ;
#8968=FACE_OUTER_BOUND ( 'NONE', #6556, .T. ) ;
#8976=EDGE_CURVE ( 'NONE', #14732, #3716, #5630, .T. ) ;
#8977=VECTOR ( 'NONE', #12811, 1000.000000000000000 ) ;
#8979=CARTESIAN_POINT ( 'NONE',  ( -7.869520639128047002, 9.000000000000001776, 0.000000000000000000 ) ) ;
#8980=LINE ( 'NONE', #7422, #5112 ) ;
#8982=LINE ( 'NONE', #4269, #7360 ) ;
#8989=CARTESIAN_POINT ( 'NONE',  ( -0.1250000000000035805, 4.999999999999999112, 1.000000000000000000 ) ) ;
#8991=LINE ( 'NONE', #10662, #6421 ) ;
#8997=EDGE_LOOP ( 'NONE', ( #20070, #13639, #2196, #2103 ) ) ;
#8998=EDGE_LOOP ( 'NONE', ( #9241, #13051, #19723, #13468 ) ) ;
#9002=ORIENTED_EDGE ( 'NONE', *, *, #16904, .T. ) ;
#9003=DIRECTION ( 'NONE',  ( 0.000000000000000000, 1.000000000000000000, -0.000000000000000000 ) ) ;
#9007=ADVANCED_FACE ( 'NONE', ( #15148 ), #6053, .F. ) ;
#9008=LINE ( 'NONE', #7544, #1842 ) ;
#9012=LINE ( 'NONE', #18323, #6721 ) ;
#9016=VECTOR ( 'NONE', #19519, 1000.000000000000114 ) ;
#9021=VERTEX_POINT ( 'NONE', #7614 ) ;
#9026=VERTEX_POINT ( 'NONE', #8778 ) ;
#9028=VECTOR ( 'NONE', #847, 1000.000000000000000 ) ;
#9029=CARTESIAN_POINT ( 'NONE',  ( -26.04469207716615031, 9.000000000000001776, 1.000000000000000000 ) ) ;
#9030=EDGE_CURVE ( 'NONE', #19766, #9549, #2387, .T. ) ;
#9036=CARTESIAN_POINT ( 'NONE',  ( -0.1250000000000035805, 9.000000000000000000, 0.000000000000000000 ) ) ;
#9041=VERTEX_POINT ( 'NONE', #16711 ) ;
#9044=FACE_OUTER_BOUND ( 'NONE', #2026, .T. ) ;
#9049=VERTEX_POINT ( 'NONE', #18290 ) ;
#9057=DIRECTION ( 'NONE',  ( 1.000000000000000000, 0.000000000000000000, 0.000000000000000000 ) ) ;
#9059=VERTEX_POINT ( 'NONE', #7518 ) ;
#9062=VECTOR ( 'NONE', #11647, 1000.000000000000000 ) ;
#9067=CARTESIAN_POINT ( 'NONE',  ( 19.73630159782011617, 4.999999999999999112, 0.000000000000000000 ) ) ;
#9068=LINE ( 'NONE', #8955, #8048 ) ;
#9075=ORIENTED_EDGE ( 'NONE', *, *, #12942, .F. ) ;
#9081=CARTESIAN_POINT ( 'NONE',  ( 0.000000000000000000, 4.999999999999999112, 1.000000000000000000 ) ) ;
#9082=VERTEX_POINT ( 'NONE', #13981 ) ;
#9086=DIRECTION ( 'NONE',  ( -0.4999999999999950040, 0.8660254037844415942, 0.000000000000000000 ) ) ;
#9104=CARTESIAN_POINT ( 'NONE',  ( 17.30017143803810242, 9.000000000000001776, 1.000000000000000000 ) ) ;
#9110=ORIENTED_EDGE ( 'NONE', *, *, #13948, .F. ) ;
#9137=CARTESIAN_POINT ( 'NONE',  ( 0.000000000000000000, 9.000000000000001776, 1.000000000000000000 ) ) ;
#9139=CARTESIAN_POINT ( 'NONE',  ( 11.99178095869207006, 0.000000000000000000, 1.000000000000000000 ) ) ;
#9146=ADVANCED_FACE ( 'NONE', ( #919 ), #7306, .T. ) ;
#9154=ORIENTED_EDGE ( 'NONE', *, *, #16928, .T. ) ;
#9156=ORIENTED_EDGE ( 'NONE', *, *, #7798, .T. ) ;
#9167=CARTESIAN_POINT ( 'NONE',  ( 21.17243175760212637, 4.999999999999999112, 1.000000000000000000 ) ) ;
#9168=CARTESIAN_POINT ( 'NONE',  ( 27.50000000000000711, 4.999999999999999112, 0.000000000000000000 ) ) ;
#9175=LINE ( 'NONE', #12820, #7374 ) ;
#9177=FACE_OUTER_BOUND ( 'NONE', #5546, .T. ) ;
#9178=ORIENTED_EDGE ( 'NONE', *, *, #7355, .T. ) ;
#9180=VERTEX_POINT ( 'NONE', #2590 ) ;
#9181=LINE ( 'NONE', #10864, #5298 ) ;
#9187=DIRECTION ( 'NONE',  ( 0.000000000000000000, -0.000000000000000000, 1.000000000000000000 ) ) ;
#9189=DIRECTION ( 'NONE',  ( 0.000000000000000000, -1.000000000000000000, 0.000000000000000000 ) ) ;
#9199=ORIENTED_EDGE ( 'NONE', *, *, #10142, .T. ) ;
#9201=VECTOR ( 'NONE', #9421, 1000.000000000000000 ) ;
#9203=VECTOR ( 'NONE', #16970, 1000.000000000000000 ) ;
#9205=ORIENTED_EDGE ( 'NONE', *, *, #19788, .F. ) ;
#9210=DIRECTION ( 'NONE',  ( 1.000000000000000000, 0.000000000000000000, 0.000000000000000000 ) ) ;
#9212=ADVANCED_FACE ( 'NONE', ( #179 ), #7920, .T. ) ;
#9222=ORIENTED_EDGE ( 'NONE', *, *, #9030, .T. ) ;
#9226=ORIENTED_EDGE ( 'NONE', *, *, #5357, .T. ) ;
#9232=EDGE_CURVE ( 'NONE', #16322, #4631, #9493, .T. ) ;
#9233=PLANE ( 'NONE',  #714 ) ;
#9234=DIRECTION ( 'NONE',  ( 0.000000000000000000, -1.000000000000000000, 0.000000000000000000 ) ) ;
#9235=CARTESIAN_POINT ( 'NONE',  ( 0.000000000000000000, 4.999999999999999112, 1.000000000000000000 ) ) ;
#9236=LINE ( 'NONE', #9139, #3382 ) ;
#9241=ORIENTED_EDGE ( 'NONE', *, *, #8447, .F. ) ;
#9247=VERTEX_POINT ( 'NONE', #11260 ) ;
#9249=CARTESIAN_POINT ( 'NONE',  ( -13.67791111847408025, 9.000000000000001776, 0.000000000000000000 ) ) ;
#9252=CARTESIAN_POINT ( 'NONE',  ( -21.42243175760212637, 0.000000000000000000, 0.000000000000000000 ) ) ;
#9258=DIRECTION ( 'NONE',  ( 0.000000000000000000, 1.000000000000000000, -0.000000000000000000 ) ) ;
#9261=LINE ( 'NONE', #8950, #20021 ) ;
#9267=DIRECTION ( 'NONE',  ( -0.000000000000000000, -0.000000000000000000, -1.000000000000000000 ) ) ;
#9275=ORIENTED_EDGE ( 'NONE', *, *, #6410, .F. ) ;
#9278=ORIENTED_EDGE ( 'NONE', *, *, #5646, .T. ) ;
#9282=CARTESIAN_POINT ( 'NONE',  ( -7.869520639128047002, 0.000000000000000000, 1.000000000000000000 ) ) ;
#9283=ADVANCED_FACE ( 'NONE', ( #1344 ), #11168, .T. ) ;
#9289=CARTESIAN_POINT ( 'NONE',  ( 21.17243175760212637, 0.000000000000000000, 1.000000000000000000 ) ) ;
#9292=AXIS2_PLACEMENT_3D ( 'NONE', #16610, #10559, #20091 ) ;
#9299=ADVANCED_FACE ( 'NONE', ( #20497 ), #6245, .T. ) ;
#9304=CARTESIAN_POINT ( 'NONE',  ( 13.42791111847407848, 0.000000000000000000, 0.000000000000000000 ) ) ;
#9305=( NAMED_UNIT ( * ) SI_UNIT ( $, .STERADIAN. ) SOLID_ANGLE_UNIT ( ) );
#9307=AXIS2_PLACEMENT_3D ( 'NONE', #6134, #4247, #2792 ) ;
#9308=LINE ( 'NONE', #8159, #5788 ) ;
#9320=CARTESIAN_POINT ( 'NONE',  ( 0.000000000000000000, 9.000000000000001776, 0.000000000000000000 ) ) ;
#9324=ORIENTED_EDGE ( 'NONE', *, *, #14510, .F. ) ;
#9327=ORIENTED_EDGE ( 'NONE', *, *, #17304, .T. ) ;
#9329=ORIENTED_EDGE ( 'NONE', *, *, #12776, .F. ) ;
#9330=FACE_OUTER_BOUND ( 'NONE', #7294, .T. ) ;
#9333=VECTOR ( 'NONE', #18083, 1000.000000000000000 ) ;
#9336=DIRECTION ( 'NONE',  ( 1.000000000000000000, 0.000000000000000000, 0.000000000000000000 ) ) ;
#9337=DIRECTION ( 'NONE',  ( 0.000000000000000000, 1.000000000000000000, 0.000000000000000000 ) ) ;
#9339=DIRECTION ( 'NONE',  ( 0.000000000000000000, 0.000000000000000000, 1.000000000000000000 ) ) ;
#9345=CARTESIAN_POINT ( 'NONE',  ( -20.00000000000000000, 0.000000000000000000, 0.5000000000000000000 ) ) ;
#9348=VECTOR ( 'NONE', #14443, 1000.000000000000000 ) ;
#9351=LINE ( 'NONE', #19093, #8389 ) ;
#9354=AXIS2_PLACEMENT_3D ( 'NONE', #10036, #208, #8474 ) ;
#9356=ORIENTED_EDGE ( 'NONE', *, *, #9874, .F. ) ;
#9368=LINE ( 'NONE', #1621, #413 ) ;
#9369=AXIS2_PLACEMENT_3D ( 'NONE', #8621, #3710, #10090 ) ;
#9371=CYLINDRICAL_SURFACE ( 'NONE', #2698, 0.5000000000000000000 ) ;
#9372=LINE ( 'NONE', #3100, #18382 ) ;
#9377=ORIENTED_EDGE ( 'NONE', *, *, #11405, .F. ) ;
#9379=LINE ( 'NONE', #10857, #8339 ) ;
#9382=EDGE_CURVE ( 'NONE', #4631, #3772, #2908, .T. ) ;
#9386=VECTOR ( 'NONE', #8940, 1000.000000000000000 ) ;
#9387=AXIS2_PLACEMENT_3D ( 'NONE', #9882, #20577, #19210 ) ;
#9388=VECTOR ( 'NONE', #8926, 1000.000000000000000 ) ;
#9389=VECTOR ( 'NONE', #6844, 1000.000000000000000 ) ;
#9396=ADVANCED_FACE ( 'NONE', ( #3015 ), #15764, .T. ) ;
#9399=FILL_AREA_STYLE ('',( #20703 ) ) ;
#9406=ORIENTED_EDGE ( 'NONE', *, *, #7691, .F. ) ;
#9409=DIRECTION ( 'NONE',  ( -0.000000000000000000, 0.000000000000000000, -1.000000000000000000 ) ) ;
#9411=VERTEX_POINT ( 'NONE', #19633 ) ;
#9413=ORIENTED_EDGE ( 'NONE', *, *, #17219, .T. ) ;
#9418=VECTOR ( 'NONE', #12125, 1000.000000000000000 ) ;
#9421=DIRECTION ( 'NONE',  ( -0.000000000000000000, 1.000000000000000000, -0.000000000000000000 ) ) ;
#9424=CARTESIAN_POINT ( 'NONE',  ( -23.35856191738413656, 9.000000000000001776, 1.000000000000000000 ) ) ;
#9428=CARTESIAN_POINT ( 'NONE',  ( -13.17791111847408025, 9.000000000000001776, 1.000000000000000000 ) ) ;
#9435=ORIENTED_EDGE ( 'NONE', *, *, #4414, .F. ) ;
#9437=LINE ( 'NONE', #15810, #9442 ) ;
#9442=VECTOR ( 'NONE', #19067, 1000.000000000000000 ) ;
#9445=LINE ( 'NONE', #2647, #5197 ) ;
#9451=VERTEX_POINT ( 'NONE', #6667 ) ;
#9467=DIRECTION ( 'NONE',  ( 0.000000000000000000, -0.000000000000000000, 1.000000000000000000 ) ) ;
#9475=FACE_OUTER_BOUND ( 'NONE', #374, .T. ) ;
#9486=ORIENTED_EDGE ( 'NONE', *, *, #7079, .T. ) ;
#9491=VERTEX_POINT ( 'NONE', #13341 ) ;
#9493=LINE ( 'NONE', #12420, #2624 ) ;
#9505=ORIENTED_EDGE ( 'NONE', *, *, #11546, .T. ) ;
#9507=ORIENTED_EDGE ( 'NONE', *, *, #13111, .T. ) ;
#9509=CARTESIAN_POINT ( 'NONE',  ( 25.04469207716615031, 4.999999999999999112, 1.000000000000000000 ) ) ;
#9510=ORIENTED_EDGE ( 'NONE', *, *, #11019, .F. ) ;
#9515=DIRECTION ( 'NONE',  ( 1.000000000000000000, 0.000000000000000000, 0.000000000000000000 ) ) ;
#9519=FACE_OUTER_BOUND ( 'NONE', #6241, .T. ) ;
#9525=DIRECTION ( 'NONE',  ( 0.000000000000000000, 1.000000000000000000, 0.000000000000000000 ) ) ;
#9526=VECTOR ( 'NONE', #9258, 1000.000000000000000 ) ;
#9529=ORIENTED_EDGE ( 'NONE', *, *, #12324, .F. ) ;
#9531=DIRECTION ( 'NONE',  ( -1.000000000000000000, 0.000000000000000000, 0.000000000000000000 ) ) ;
#9533=EDGE_CURVE ( 'NONE', #15883, #19, #19743, .T. ) ;
#9535=PLANE ( 'NONE',  #10450 ) ;
#9538=AXIS2_PLACEMENT_3D ( 'NONE', #495, #3431, #9808 ) ;
#9541=EDGE_CURVE ( 'NONE', #6861, #5289, #8540, .T. ) ;
#9549=VERTEX_POINT ( 'NONE', #9802 ) ;
#9562=DIRECTION ( 'NONE',  ( -1.000000000000000000, -1.734723475976807094E-15, 0.000000000000000000 ) ) ;
#9563=EDGE_LOOP ( 'NONE', ( #1082, #5599, #9997, #76 ) ) ;
#9565=CARTESIAN_POINT ( 'NONE',  ( 11.99178095869207006, 0.000000000000000000, 0.000000000000000000 ) ) ;
#9568=LINE ( 'NONE', #20575, #15768 ) ;
#9569=CARTESIAN_POINT ( 'NONE',  ( 21.67243175760212637, 4.999999999999999112, 1.000000000000000000 ) ) ;
#9570=DIRECTION ( 'NONE',  ( -1.000000000000000000, 0.000000000000000000, 0.000000000000000000 ) ) ;
#9571=DIRECTION ( 'NONE',  ( 0.000000000000000000, -1.000000000000000000, 0.000000000000000000 ) ) ;
#9580=ORIENTED_EDGE ( 'NONE', *, *, #8154, .T. ) ;
#9581=ORIENTED_EDGE ( 'NONE', *, *, #10655, .T. ) ;
#9583=VERTEX_POINT ( 'NONE', #5095 ) ;
#9585=EDGE_CURVE ( 'NONE', #14879, #14595, #1117, .T. ) ;
#9586=ORIENTED_EDGE ( 'NONE', *, *, #15537, .F. ) ;
#9592=DIRECTION ( 'NONE',  ( 0.000000000000000000, 1.000000000000000000, -0.000000000000000000 ) ) ;
#9598=LINE ( 'NONE', #12740, #15756 ) ;
#9600=VERTEX_POINT ( 'NONE', #15124 ) ;
#9603=ORIENTED_EDGE ( 'NONE', *, *, #2244, .F. ) ;
#9604=CARTESIAN_POINT ( 'NONE',  ( 13.00000000000000355, 7.806255641895631925E-15, 2.000000000000000000 ) ) ;
#9608=VERTEX_POINT ( 'NONE', #13546 ) ;
#9611=EDGE_CURVE ( 'NONE', #12804, #20155, #3929, .T. ) ;
#9612=CARTESIAN_POINT ( 'NONE',  ( 0.000000000000000000, 9.000000000000001776, 1.000000000000000000 ) ) ;
#9616=LINE ( 'NONE', #8065, #12351 ) ;
#9629=VECTOR ( 'NONE', #8563, 1000.000000000000000 ) ;
#9631=VERTEX_POINT ( 'NONE', #7282 ) ;
#9635=DIRECTION ( 'NONE',  ( 1.000000000000000000, 0.000000000000000000, 0.000000000000000000 ) ) ;
#9644=LINE ( 'NONE', #12782, #15099 ) ;
#9645=CARTESIAN_POINT ( 'NONE',  ( -3.999999999999999112, -2.500000000000047518, 2.000000000000000000 ) ) ;
#9655=EDGE_LOOP ( 'NONE', ( #2328, #18050, #2947, #18939 ) ) ;
#9666=DIRECTION ( 'NONE',  ( 0.000000000000000000, 0.000000000000000000, 1.000000000000000000 ) ) ;
#9673=EDGE_CURVE ( 'NONE', #19645, #18629, #18682, .T. ) ;
#9674=CARTESIAN_POINT ( 'NONE',  ( -27.52582389412042474, 4.853545418763153485, 0.000000000000000000 ) ) ;
#9676=CARTESIAN_POINT ( 'NONE',  ( 5.683390479346035029, 0.000000000000000000, 1.000000000000000000 ) ) ;
#9677=CARTESIAN_POINT ( 'NONE',  ( 0.3749999999999968914, 4.999999999999999112, 1.000000000000000000 ) ) ;
#9682=AXIS2_PLACEMENT_3D ( 'NONE', #516, #1982, #19664 ) ;
#9684=EDGE_LOOP ( 'NONE', ( #8161, #13691, #715, #5181 ) ) ;
#9688=VERTEX_POINT ( 'NONE', #4349 ) ;
#9689=CARTESIAN_POINT ( 'NONE',  ( 0.000000000000000000, 4.999999999999999112, 1.000000000000000000 ) ) ;
#9690=ORIENTED_EDGE ( 'NONE', *, *, #19019, .T. ) ;
#9692=VECTOR ( 'NONE', #18791, 1000.000000000000000 ) ;
#9694=VERTEX_POINT ( 'NONE', #19850 ) ;
#9697=VECTOR ( 'NONE', #17835, 1000.000000000000000 ) ;
#9708=DIRECTION ( 'NONE',  ( -0.000000000000000000, -0.000000000000000000, -1.000000000000000000 ) ) ;
#9710=ORIENTED_EDGE ( 'NONE', *, *, #16136, .F. ) ;
#9712=VECTOR ( 'NONE', #5078, 1000.000000000000000 ) ;
#9714=LINE ( 'NONE', #1768, #5992 ) ;
#9723=PLANE ( 'NONE',  #12790 ) ;
#9725=VECTOR ( 'NONE', #7034, 1000.000000000000000 ) ;
#9732=ADVANCED_FACE ( 'NONE', ( #10524 ), #800, .T. ) ;
#9738=EDGE_LOOP ( 'NONE', ( #20299, #17688, #4798, #10770 ) ) ;
#9741=EDGE_CURVE ( 'NONE', #7048, #10510, #15321, .T. ) ;
#9743=DIRECTION ( 'NONE',  ( -0.000000000000000000, -0.000000000000000000, -1.000000000000000000 ) ) ;
#9744=ORIENTED_EDGE ( 'NONE', *, *, #18430, .F. ) ;
#9747=DIRECTION ( 'NONE',  ( -0.000000000000000000, -0.000000000000000000, -1.000000000000000000 ) ) ;
#9760=ORIENTED_EDGE ( 'NONE', *, *, #3902, .T. ) ;
#9762=CARTESIAN_POINT ( 'NONE',  ( 17.30017143803810242, 9.000000000000001776, 1.000000000000000000 ) ) ;
#9772=DIRECTION ( 'NONE',  ( 1.000000000000000000, 0.000000000000000000, 0.000000000000000000 ) ) ;
#9778=DIRECTION ( 'NONE',  ( -1.000000000000000000, 0.000000000000000000, 0.000000000000000000 ) ) ;
#9782=LINE ( 'NONE', #19110, #8977 ) ;
#9800=ORIENTED_EDGE ( 'NONE', *, *, #15724, .T. ) ;
#9802=CARTESIAN_POINT ( 'NONE',  ( -13.17791111847408025, 9.000000000000001776, 1.000000000000000000 ) ) ;
#9808=DIRECTION ( 'NONE',  ( -0.000000000000000000, 0.000000000000000000, -1.000000000000000000 ) ) ;
#9816=LINE ( 'NONE', #13156, #16959 ) ;
#9817=DIRECTION ( 'NONE',  ( 0.000000000000000000, 1.000000000000000000, -0.000000000000000000 ) ) ;
#9818=ORIENTED_EDGE ( 'NONE', *, *, #12618, .T. ) ;
#9820=ORIENTED_EDGE ( 'NONE', *, *, #13005, .F. ) ;
#9834=DIRECTION ( 'NONE',  ( 1.000000000000000000, 0.000000000000000000, 0.000000000000000000 ) ) ;
#9835=DIRECTION ( 'NONE',  ( -0.000000000000000000, -0.000000000000000000, -1.000000000000000000 ) ) ;
#9839=ORIENTED_EDGE ( 'NONE', *, *, #12578, .F. ) ;
#9843=ORIENTED_EDGE ( 'NONE', *, *, #7331, .T. ) ;
#9845=LINE ( 'NONE', #13279, #11118 ) ;
#9847=EDGE_CURVE ( 'NONE', #17893, #16449, #1420, .T. ) ;
#9850=DIRECTION ( 'NONE',  ( -0.000000000000000000, -0.000000000000000000, -1.000000000000000000 ) ) ;
#9860=VECTOR ( 'NONE', #13759, 1000.000000000000000 ) ;
#9863=EDGE_LOOP ( 'NONE', ( #8510, #14195, #14703, #19082 ) ) ;
#9868=ORIENTED_EDGE ( 'NONE', *, *, #19526, .T. ) ;
#9869=CARTESIAN_POINT ( 'NONE',  ( -4.999999999999998224, -7.500000000000047073, 9.999999999999998224 ) ) ;
#9874=EDGE_CURVE ( 'NONE', #17197, #9600, #53, .T. ) ;
#9878=EDGE_CURVE ( 'NONE', #5573, #15088, #20667, .T. ) ;
#9879=CARTESIAN_POINT ( 'NONE',  ( 0.000000000000000000, 0.000000000000000000, 1.000000000000000000 ) ) ;
#9882=CARTESIAN_POINT ( 'NONE',  ( -11.74178095869206828, 0.000000000000000000, 1.000000000000000000 ) ) ;
#9887=EDGE_CURVE ( 'NONE', #8074, #20271, #7897, .T. ) ;
#9897=PLANE ( 'NONE',  #4086 ) ;
#9899=VERTEX_POINT ( 'NONE', #15530 ) ;
#9900=LINE ( 'NONE', #19849, #6997 ) ;
#9907=PLANE ( 'NONE',  #9538 ) ;
#9917=DIRECTION ( 'NONE',  ( 0.000000000000000000, -0.000000000000000000, 1.000000000000000000 ) ) ;
#9919=ORIENTED_EDGE ( 'NONE', *, *, #20354, .F. ) ;
#9924=DIRECTION ( 'NONE',  ( -0.000000000000000000, -0.000000000000000000, -1.000000000000000000 ) ) ;
#9926=CARTESIAN_POINT ( 'NONE',  ( -3.999999999999999112, -7.500000000000047073, 2.000000000000000000 ) ) ;
#9929=DIRECTION ( 'NONE',  ( 1.000000000000000000, 0.000000000000000000, 0.000000000000000000 ) ) ;
#9940=ORIENTED_EDGE ( 'NONE', *, *, #1874, .T. ) ;
#9943=PLANE ( 'NONE',  #13429 ) ;
#9947=DIRECTION ( 'NONE',  ( 1.000000000000000000, 0.000000000000000000, 0.000000000000000000 ) ) ;
#9949=DIRECTION ( 'NONE',  ( -0.000000000000000000, -0.000000000000000000, -1.000000000000000000 ) ) ;
#9954=LINE ( 'NONE', #5462, #19103 ) ;
#9960=DIRECTION ( 'NONE',  ( 1.000000000000000000, 0.000000000000000000, 0.000000000000000000 ) ) ;
#9968=ORIENTED_EDGE ( 'NONE', *, *, #7515, .T. ) ;
#9971=AXIS2_PLACEMENT_3D ( 'NONE', #3502, #16263, #17422 ) ;
#9977=CARTESIAN_POINT ( 'NONE',  ( -2.061130159782011972, 0.000000000000000000, 0.000000000000000000 ) ) ;
#9978=CARTESIAN_POINT ( 'NONE',  ( 0.000000000000000000, 9.000000000000001776, 1.000000000000000000 ) ) ;
#9980=LINE ( 'NONE', #13424, #5978 ) ;
#9985=ORIENTED_EDGE ( 'NONE', *, *, #18074, .T. ) ;
#9988=ADVANCED_FACE ( 'NONE', ( #11015 ), #3372, .T. ) ;
#9994=EDGE_LOOP ( 'NONE', ( #16422, #13254, #3277, #15345 ) ) ;
#9996=CARTESIAN_POINT ( 'NONE',  ( -11.24178095869206828, 9.000000000000001776, 0.000000000000000000 ) ) ;
#9997=ORIENTED_EDGE ( 'NONE', *, *, #4034, .T. ) ;
#9998=CARTESIAN_POINT ( 'NONE',  ( 8.119520639128047890, 0.000000000000000000, 0.000000000000000000 ) ) ;
#10005=VECTOR ( 'NONE', #3085, 1000.000000000000000 ) ;
#10009=CARTESIAN_POINT ( 'NONE',  ( 0.000000000000000000, 9.000000000000001776, 1.000000000000000000 ) ) ;
#10011=CARTESIAN_POINT ( 'NONE',  ( -17.55017143803810242, 0.000000000000000000, 0.000000000000000000 ) ) ;
#10015=ORIENTED_EDGE ( 'NONE', *, *, #1394, .F. ) ;
#10020=DIRECTION ( 'NONE',  ( -1.734723475976807094E-15, -1.000000000000000000, 0.000000000000000000 ) ) ;
#10033=VECTOR ( 'NONE', #13783, 1000.000000000000000 ) ;
#10036=CARTESIAN_POINT ( 'NONE',  ( -27.52582389412042474, 4.853545418763153485, 1.000000000000000000 ) ) ;
#10039=VECTOR ( 'NONE', #6136, 1000.000000000000000 ) ;
#10045=CARTESIAN_POINT ( 'NONE',  ( 0.3749999999999968914, 4.999999999999999112, 0.000000000000000000 ) ) ;
#10048=VERTEX_POINT ( 'NONE', #14342 ) ;
#10049=ADVANCED_FACE ( 'NONE', ( #26 ), #19181, .T. ) ;
#10056=CARTESIAN_POINT ( 'NONE',  ( -20.00000000000000000, -6.000000000000000000, 2.000000000000000000 ) ) ;
#10057=AXIS2_PLACEMENT_3D ( 'NONE', #10830, #20562, #18669 ) ;
#10059=DIRECTION ( 'NONE',  ( 1.000000000000000000, 0.000000000000000000, 0.000000000000000000 ) ) ;
#10060=VECTOR ( 'NONE', #9960, 1000.000000000000000 ) ;
#10062=VECTOR ( 'NONE', #12143, 1000.000000000000000 ) ;
#10068=CARTESIAN_POINT ( 'NONE',  ( -15.61404127825609223, 4.999999999999999112, 0.000000000000000000 ) ) ;
#10075=EDGE_LOOP ( 'NONE', ( #15978, #9324, #19241, #14599 ) ) ;
#10086=CARTESIAN_POINT ( 'NONE',  ( -18.98630159782011262, 4.999999999999999112, 1.000000000000000000 ) ) ;
#10088=CARTESIAN_POINT ( 'NONE',  ( 20.00000000000000000, 3.000000000000004441, 2.000000000000000000 ) ) ;
#10090=DIRECTION ( 'NONE',  ( 0.000000000000000000, -0.000000000000000000, -1.000000000000000000 ) ) ;
#10094=EDGE_LOOP ( 'NONE', ( #15339, #7513, #9156, #17709 ) ) ;
#10100=VERTEX_POINT ( 'NONE', #10235 ) ;
#10113=CARTESIAN_POINT ( 'NONE',  ( 0.000000000000000000, 4.999999999999999112, 0.000000000000000000 ) ) ;
#10114=VECTOR ( 'NONE', #19708, 1000.000000000000000 ) ;
#10126=ORIENTED_EDGE ( 'NONE', *, *, #8886, .F. ) ;
#10128=CARTESIAN_POINT ( 'NONE',  ( -15.11404127825609223, 4.999999999999999112, 1.000000000000000000 ) ) ;
#10129=ORIENTED_EDGE ( 'NONE', *, *, #10578, .F. ) ;
#10130=ORIENTED_EDGE ( 'NONE', *, *, #18205, .T. ) ;
#10133=ORIENTED_EDGE ( 'NONE', *, *, #11895, .T. ) ;
#10136=ADVANCED_FACE ( 'NONE', ( #12217 ), #10550, .F. ) ;
#10138=DIRECTION ( 'NONE',  ( 1.000000000000000000, 0.000000000000000000, -0.000000000000000000 ) ) ;
#10142=EDGE_CURVE ( 'NONE', #3140, #6097, #7209, .T. ) ;
#10152=ORIENTED_EDGE ( 'NONE', *, *, #18519, .F. ) ;
#10155=ORIENTED_EDGE ( 'NONE', *, *, #3876, .T. ) ;
#10156=LINE ( 'NONE', #17802, #3442 ) ;
#10158=DIRECTION ( 'NONE',  ( 0.000000000000000000, -0.000000000000000000, 1.000000000000000000 ) ) ;
#10159=LINE ( 'NONE', #19897, #12985 ) ;
#10161=EDGE_CURVE ( 'NONE', #12873, #8157, #4067, .T. ) ;
#10167=CARTESIAN_POINT ( 'NONE',  ( -5.999999999999999112, -2.500000000000047518, 9.999999999999998224 ) ) ;
#10168=CARTESIAN_POINT ( 'NONE',  ( 0.000000000000000000, 9.000000000000001776, 0.000000000000000000 ) ) ;
#10179=ORIENTED_EDGE ( 'NONE', *, *, #7884, .T. ) ;
#10182=ADVANCED_FACE ( 'NONE', ( #16823 ), #19875, .T. ) ;
#10188=LINE ( 'NONE', #8730, #5056 ) ;
#10190=CARTESIAN_POINT ( 'NONE',  ( -17.11324865405191176, -11.00000000000000000, 2.000000000000000000 ) ) ;
#10200=VECTOR ( 'NONE', #18218, 1000.000000000000000 ) ;
#10201=CARTESIAN_POINT ( 'NONE',  ( -24.50000000000000000, 0.000000000000000000, 1.000000000000000000 ) ) ;
#10202=ORIENTED_EDGE ( 'NONE', *, *, #19635, .F. ) ;
#10203=AXIS2_PLACEMENT_3D ( 'NONE', #15713, #4324, #5892 ) ;
#10206=ORIENTED_EDGE ( 'NONE', *, *, #18743, .T. ) ;
#10207=LINE ( 'NONE', #9998, #3415 ) ;
#10220=ORIENTED_EDGE ( 'NONE', *, *, #12428, .F. ) ;
#10225=LINE ( 'NONE', #8353, #18979 ) ;
#10232=CARTESIAN_POINT ( 'NONE',  ( 5.999999999999999112, -7.500000000000047073, 2.000000000000000000 ) ) ;
#10235=CARTESIAN_POINT ( 'NONE',  ( -17.55017143803810242, 4.999999999999999112, 1.000000000000000000 ) ) ;
#10237=CARTESIAN_POINT ( 'NONE',  ( -24.50000000000000000, 3.000000000000000888, 1.000000000000000000 ) ) ;
#10243=PLANE ( 'NONE',  #9292 ) ;
#10249=VERTEX_POINT ( 'NONE', #8979 ) ;
#10251=LINE ( 'NONE', #5138, #2091 ) ;
#10257=EDGE_CURVE ( 'NONE', #7202, #5157, #16713, .T. ) ;
#10259=CARTESIAN_POINT ( 'NONE',  ( 0.000000000000000000, 9.000000000000001776, 0.000000000000000000 ) ) ;
#10266=DIRECTION ( 'NONE',  ( 0.000000000000000000, 1.000000000000000000, 0.000000000000000000 ) ) ;
#10268=CARTESIAN_POINT ( 'NONE',  ( 19.73630159782011617, 9.000000000000001776, 0.000000000000000000 ) ) ;
#10270=EDGE_CURVE ( 'NONE', #7916, #10336, #5848, .T. ) ;
#10273=ORIENTED_EDGE ( 'NONE', *, *, #8645, .T. ) ;
#10282=AXIS2_PLACEMENT_3D ( 'NONE', #10451, #4375, #9086 ) ;
#10285=LINE ( 'NONE', #18243, #14995 ) ;
#10287=CARTESIAN_POINT ( 'NONE',  ( 5.999999999999999112, -2.500000000000047518, 2.000000000000000000 ) ) ;
#10288=CARTESIAN_POINT ( 'NONE',  ( -13.67791111847408025, 4.999999999999999112, 1.000000000000000000 ) ) ;
#10289=VECTOR ( 'NONE', #13773, 1000.000000000000000 ) ;
#10294=EDGE_LOOP ( 'NONE', ( #10807, #12388, #18161, #19754 ) ) ;
#10300=ORIENTED_EDGE ( 'NONE', *, *, #3366, .T. ) ;
#10304=ORIENTED_EDGE ( 'NONE', *, *, #2725, .T. ) ;
#10307=DIRECTION ( 'NONE',  ( -0.000000000000000000, -0.000000000000000000, -1.000000000000000000 ) ) ;
#10309=ORIENTED_EDGE ( 'NONE', *, *, #17569, .T. ) ;
#10314=DIRECTION ( 'NONE',  ( 1.000000000000000000, 0.000000000000000000, 0.000000000000000000 ) ) ;
#10315=DIRECTION ( 'NONE',  ( 1.000000000000000000, 0.000000000000000000, 0.000000000000000000 ) ) ;
#10316=VECTOR ( 'NONE', #10315, 1000.000000000000000 ) ;
#10323=AXIS2_PLACEMENT_3D ( 'NONE', #15557, #1237, #1343 ) ;
#10328=ORIENTED_EDGE ( 'NONE', *, *, #11845, .F. ) ;
#10331=EDGE_LOOP ( 'NONE', ( #3589, #4036, #6124, #15992 ) ) ;
#10333=CARTESIAN_POINT ( 'NONE',  ( -26.79469207716615387, 9.000000000000001776, 1.000000000000000000 ) ) ;
#10336=VERTEX_POINT ( 'NONE', #12621 ) ;
#10345=CARTESIAN_POINT ( 'NONE',  ( 19.23630159782011617, 0.000000000000000000, 1.000000000000000000 ) ) ;
#10346=LINE ( 'NONE', #15460, #13023 ) ;
#10351=VERTEX_POINT ( 'NONE', #14189 ) ;
#10359=ORIENTED_EDGE ( 'NONE', *, *, #14456, .F. ) ;
#10361=LINE ( 'NONE', #632, #5422 ) ;
#10363=DIRECTION ( 'NONE',  ( -0.000000000000000000, -0.000000000000000000, -1.000000000000000000 ) ) ;
#10364=CARTESIAN_POINT ( 'NONE',  ( 20.00000000000000000, 3.000000000000004441, 1.000000000000000000 ) ) ;
#10368=CARTESIAN_POINT ( 'NONE',  ( 0.3749999999999968914, 0.000000000000000000, 1.000000000000000000 ) ) ;
#10370=AXIS2_PLACEMENT_3D ( 'NONE', #11721, #19896, #10158 ) ;
#10371=ADVANCED_FACE ( 'NONE', ( #15766 ), #6055, .T. ) ;
#10374=LINE ( 'NONE', #9289, #8858 ) ;
#10377=PLANE ( 'NONE',  #5697 ) ;
#10378=EDGE_CURVE ( 'NONE', #1315, #7476, #1544, .T. ) ;
#10383=DIRECTION ( 'NONE',  ( -1.000000000000000000, 0.000000000000000000, 0.000000000000000000 ) ) ;
#10389=ORIENTED_EDGE ( 'NONE', *, *, #9611, .T. ) ;
#10390=VECTOR ( 'NONE', #8618, 1000.000000000000000 ) ;
#10391=VECTOR ( 'NONE', #13909, 1000.000000000000000 ) ;
#10392=VERTEX_POINT ( 'NONE', #14091 ) ;
#10397=DIRECTION ( 'NONE',  ( 1.000000000000000000, 0.000000000000000000, 0.000000000000000000 ) ) ;
#10399=DIRECTION ( 'NONE',  ( 1.000000000000000000, 0.000000000000000000, 0.000000000000000000 ) ) ;
#10405=ORIENTED_EDGE ( 'NONE', *, *, #5858, .T. ) ;
#10410=ORIENTED_EDGE ( 'NONE', *, *, #12211, .T. ) ;
#10413=ORIENTED_EDGE ( 'NONE', *, *, #8488, .T. ) ;
#10416=DIRECTION ( 'NONE',  ( 0.000000000000000000, -1.000000000000000000, 0.000000000000000000 ) ) ;
#10422=EDGE_LOOP ( 'NONE', ( #7659, #10493, #2201, #19188, #2721, #4725 ) ) ;
#10427=CARTESIAN_POINT ( 'NONE',  ( 11.49178095869207006, 4.999999999999999112, 0.000000000000000000 ) ) ;
#10431=LINE ( 'NONE', #8648, #12969 ) ;
#10450=AXIS2_PLACEMENT_3D ( 'NONE', #8183, #6609, #12978 ) ;
#10451=CARTESIAN_POINT ( 'NONE',  ( -20.00000000000000000, -6.000000000000000000, 2.000000000000000000 ) ) ;
#10452=ADVANCED_FACE ( 'NONE', ( #15663 ), #1347, .T. ) ;
#10454=CARTESIAN_POINT ( 'NONE',  ( 0.000000000000000000, 4.999999999999999112, 0.000000000000000000 ) ) ;
#10460=ORIENTED_EDGE ( 'NONE', *, *, #11530, .T. ) ;
#10461=CARTESIAN_POINT ( 'NONE',  ( -11.74178095869206828, 9.000000000000001776, 1.000000000000000000 ) ) ;
#10462=CARTESIAN_POINT ( 'NONE',  ( 27.50000000000000711, 4.999999999999999112, 1.000000000000000000 ) ) ;
#10465=EDGE_CURVE ( 'NONE', #13688, #6649, #278, .T. ) ;
#10467=DIRECTION ( 'NONE',  ( 1.000000000000000000, 0.000000000000000000, -0.000000000000000000 ) ) ;
#10468=EDGE_LOOP ( 'NONE', ( #202, #13663, #476, #894 ) ) ;
#10469=ORIENTED_EDGE ( 'NONE', *, *, #2217, .T. ) ;
#10477=FACE_OUTER_BOUND ( 'NONE', #20717, .T. ) ;
#10483=LINE ( 'NONE', #5563, #4035 ) ;
#10493=ORIENTED_EDGE ( 'NONE', *, *, #6171, .T. ) ;
#10497=CARTESIAN_POINT ( 'NONE',  ( -17.05017143803810242, 4.999999999999999112, 1.000000000000000000 ) ) ;
#10498=DIRECTION ( 'NONE',  ( -0.1736481776669295540, 0.9848077530122082424, 0.000000000000000000 ) ) ;
#10501=DIRECTION ( 'NONE',  ( 0.000000000000000000, -0.000000000000000000, 1.000000000000000000 ) ) ;
#10505=EDGE_LOOP ( 'NONE', ( #3184, #17155 ) ) ;
#10507=LINE ( 'NONE', #14150, #16400 ) ;
#10510=VERTEX_POINT ( 'NONE', #3623 ) ;
#10514=ORIENTED_EDGE ( 'NONE', *, *, #3222, .F. ) ;
#10515=CARTESIAN_POINT ( 'NONE',  ( 27.50000000000000711, 4.999999999999999112, 1.000000000000000000 ) ) ;
#10517=ORIENTED_EDGE ( 'NONE', *, *, #5845, .T. ) ;
#10519=CIRCLE ( 'NONE', #18539, 2.999999999999999112 ) ;
#10523=CARTESIAN_POINT ( 'NONE',  ( -3.497260319564023057, 0.000000000000000000, 1.000000000000000000 ) ) ;
#10524=FACE_OUTER_BOUND ( 'NONE', #8771, .T. ) ;
#10529=CARTESIAN_POINT ( 'NONE',  ( 0.000000000000000000, 4.999999999999999112, 0.000000000000000000 ) ) ;
#10531=CARTESIAN_POINT ( 'NONE',  ( -20.92243175760212637, 9.000000000000001776, 1.000000000000000000 ) ) ;
#10540=LINE ( 'NONE', #2583, #15630 ) ;
#10545=ORIENTED_EDGE ( 'NONE', *, *, #10465, .F. ) ;
#10547=DIRECTION ( 'NONE',  ( 1.000000000000000000, 0.000000000000000000, 0.000000000000000000 ) ) ;
#10550=PLANE ( 'NONE',  #16379 ) ;
#10558=ORIENTED_EDGE ( 'NONE', *, *, #6560, .T. ) ;
#10559=DIRECTION ( 'NONE',  ( -0.7071067811865475727, 0.000000000000000000, -0.7071067811865475727 ) ) ;
#10566=EDGE_LOOP ( 'NONE', ( #20565, #7278, #13560, #17898 ) ) ;
#10567=EDGE_CURVE ( 'NONE', #2846, #14519, #16385, .T. ) ;
#10572=CARTESIAN_POINT ( 'NONE',  ( 0.000000000000000000, 4.999999999999999112, 1.000000000000000000 ) ) ;
#10573=VERTEX_POINT ( 'NONE', #19332 ) ;
#10576=CARTESIAN_POINT ( 'NONE',  ( -14.00000000000000000, 0.000000000000000000, 1.000000000000000000 ) ) ;
#10578=EDGE_CURVE ( 'NONE', #2072, #3209, #2063, .T. ) ;
#10583=LINE ( 'NONE', #16751, #14708 ) ;
#10590=ORIENTED_EDGE ( 'NONE', *, *, #3150, .F. ) ;
#10591=ORIENTED_EDGE ( 'NONE', *, *, #15811, .F. ) ;
#10592=CARTESIAN_POINT ( 'NONE',  ( -0.1250000000000035805, 4.999999999999999112, 0.000000000000000000 ) ) ;
#10598=DIRECTION ( 'NONE',  ( 0.000000000000000000, 1.000000000000000000, 0.000000000000000000 ) ) ;
#10599=CARTESIAN_POINT ( 'NONE',  ( -19.48630159782011262, 9.000000000000001776, 0.000000000000000000 ) ) ;
#10603=ORIENTED_EDGE ( 'NONE', *, *, #19526, .F. ) ;
#10618=LINE ( 'NONE', #15429, #2546 ) ;
#10620=DIRECTION ( 'NONE',  ( 1.000000000000000000, 0.000000000000000000, -0.000000000000000000 ) ) ;
#10627=CARTESIAN_POINT ( 'NONE',  ( 6.183390479346035917, 4.999999999999999112, 0.000000000000000000 ) ) ;
#10629=CARTESIAN_POINT ( 'NONE',  ( 19.23630159782011617, 9.000000000000001776, 1.000000000000000000 ) ) ;
#10635=ORIENTED_EDGE ( 'NONE', *, *, #20017, .F. ) ;
#10636=EDGE_CURVE ( 'NONE', #20224, #19548, #12262, .T. ) ;
#10643=FACE_OUTER_BOUND ( 'NONE', #8437, .T. ) ;
#10644=ORIENTED_EDGE ( 'NONE', *, *, #18634, .T. ) ;
#10647=VERTEX_POINT ( 'NONE', #20233 ) ;
#10648=LINE ( 'NONE', #4064, #6658 ) ;
#10653=DIRECTION ( 'NONE',  ( 1.000000000000000000, 0.000000000000000000, 0.000000000000000000 ) ) ;
#10655=EDGE_CURVE ( 'NONE', #487, #16591, #12475, .T. ) ;
#10662=CARTESIAN_POINT ( 'NONE',  ( -5.433390479346035029, 0.000000000000000000, 0.000000000000000000 ) ) ;
#10672=AXIS2_PLACEMENT_3D ( 'NONE', #11569, #18164, #3830 ) ;
#10673=CARTESIAN_POINT ( 'NONE',  ( 0.000000000000000000, 9.000000000000001776, 1.000000000000000000 ) ) ;
#10679=CARTESIAN_POINT ( 'NONE',  ( -19.48630159782011262, 0.000000000000000000, 1.000000000000000000 ) ) ;
#10683=VECTOR ( 'NONE', #17068, 1000.000000000000000 ) ;
#10699=ADVANCED_FACE ( 'NONE', ( #18656 ), #17080, .T. ) ;
#10702=AXIS2_PLACEMENT_3D ( 'NONE', #16262, #11648, #671 ) ;
#10709=DIRECTION ( 'NONE',  ( 0.000000000000000000, 1.000000000000000000, -0.000000000000000000 ) ) ;
#10710=DIRECTION ( 'NONE',  ( 0.000000000000000000, -0.000000000000000000, 1.000000000000000000 ) ) ;
#10713=VERTEX_POINT ( 'NONE', #15605 ) ;
#10716=DIRECTION ( 'NONE',  ( -0.000000000000000000, -0.000000000000000000, -1.000000000000000000 ) ) ;
#10720=ORIENTED_EDGE ( 'NONE', *, *, #17706, .T. ) ;
#10730=AXIS2_PLACEMENT_3D ( 'NONE', #2939, #18950, #4605 ) ;
#10731=ORIENTED_EDGE ( 'NONE', *, *, #17986, .F. ) ;
#10738=CARTESIAN_POINT ( 'NONE',  ( 0.000000000000000000, 9.000000000000001776, 0.000000000000000000 ) ) ;
#10740=PLANE ( 'NONE',  #18312 ) ;
#10742=CARTESIAN_POINT ( 'NONE',  ( 21.17243175760212637, 0.000000000000000000, 0.000000000000000000 ) ) ;
#10753=EDGE_LOOP ( 'NONE', ( #10756, #12562, #2080, #5392 ) ) ;
#10755=EDGE_CURVE ( 'NONE', #3444, #1636, #6200, .T. ) ;
#10756=ORIENTED_EDGE ( 'NONE', *, *, #17673, .F. ) ;
#10757=CARTESIAN_POINT ( 'NONE',  ( 8.119520639128047890, 4.999999999999999112, 0.000000000000000000 ) ) ;
#10759=EDGE_CURVE ( 'NONE', #16591, #17, #9445, .T. ) ;
#10763=ADVANCED_FACE ( 'NONE', ( #7567 ), #12164, .T. ) ;
#10765=DIRECTION ( 'NONE',  ( 1.000000000000000000, 0.000000000000000000, 0.000000000000000000 ) ) ;
#10770=ORIENTED_EDGE ( 'NONE', *, *, #3150, .T. ) ;
#10775=VECTOR ( 'NONE', #10416, 1000.000000000000000 ) ;
#10777=CARTESIAN_POINT ( 'NONE',  ( -3.497260319564023057, 9.000000000000001776, 1.000000000000000000 ) ) ;
#10782=ORIENTED_EDGE ( 'NONE', *, *, #6489, .T. ) ;
#10783=VECTOR ( 'NONE', #12898, 1000.000000000000000 ) ;
#10784=EDGE_CURVE ( 'NONE', #2075, #2607, #7779, .T. ) ;
#10790=DIRECTION ( 'NONE',  ( 0.000000000000000000, 1.000000000000000000, 0.000000000000000000 ) ) ;
#10793=LINE ( 'NONE', #20109, #16403 ) ;
#10795=LINE ( 'NONE', #5774, #16411 ) ;
#10798=DIRECTION ( 'NONE',  ( -0.000000000000000000, -0.000000000000000000, -1.000000000000000000 ) ) ;
#10807=ORIENTED_EDGE ( 'NONE', *, *, #16617, .F. ) ;
#10809=LINE ( 'NONE', #12058, #3428 ) ;
#10810=VECTOR ( 'NONE', #18423, 1000.000000000000000 ) ;
#10814=CARTESIAN_POINT ( 'NONE',  ( -13.00000000000000355, 6.123233995736754943E-17, 2.000000000000000000 ) ) ;
#10816=CARTESIAN_POINT ( 'NONE',  ( 0.000000000000000000, 4.999999999999999112, 0.000000000000000000 ) ) ;
#10817=FACE_OUTER_BOUND ( 'NONE', #17297, .T. ) ;
#10818=EDGE_CURVE ( 'NONE', #11436, #9041, #3125, .T. ) ;
#10830=CARTESIAN_POINT ( 'NONE',  ( 26.04469207716615031, 0.000000000000000000, 1.000000000000000000 ) ) ;
#10831=ORIENTED_EDGE ( 'NONE', *, *, #5398, .F. ) ;
#10833=CARTESIAN_POINT ( 'NONE',  ( -11.74178095869206828, 9.000000000000001776, 0.000000000000000000 ) ) ;
#10835=VERTEX_POINT ( 'NONE', #19030 ) ;
#10838=VECTOR ( 'NONE', #18350, 1000.000000000000000 ) ;
#10840=ORIENTED_EDGE ( 'NONE', *, *, #13403, .T. ) ;
#10845=LINE ( 'NONE', #12401, #5965 ) ;
#10848=FACE_OUTER_BOUND ( 'NONE', #18594, .T. ) ;
#10857=CARTESIAN_POINT ( 'NONE',  ( 2.311130159782011972, 0.000000000000000000, 0.000000000000000000 ) ) ;
#10862=MANIFOLD_SOLID_BREP ( 'Chamfer1', #2975 ) ;
#10864=CARTESIAN_POINT ( 'NONE',  ( 6.183390479346035917, 0.000000000000000000, 0.000000000000000000 ) ) ;
#10874=ORIENTED_EDGE ( 'NONE', *, *, #7611, .T. ) ;
#10876=FACE_OUTER_BOUND ( 'NONE', #17744, .T. ) ;
#10881=ORIENTED_EDGE ( 'NONE', *, *, #1074, .T. ) ;
#10884=VECTOR ( 'NONE', #3069, 1000.000000000000000 ) ;
#10886=CARTESIAN_POINT ( 'NONE',  ( 27.52582389412042474, 4.853545418763153485, 1.000000000000000000 ) ) ;
#10889=DIRECTION ( 'NONE',  ( 0.000000000000000000, 1.000000000000000000, 0.000000000000000000 ) ) ;
#10906=ORIENTED_EDGE ( 'NONE', *, *, #471, .T. ) ;
#10908=CARTESIAN_POINT ( 'NONE',  ( -3.497260319564023057, 0.000000000000000000, 1.000000000000000000 ) ) ;
#10913=DIRECTION ( 'NONE',  ( 0.000000000000000000, -0.000000000000000000, 1.000000000000000000 ) ) ;
#10915=CARTESIAN_POINT ( 'NONE',  ( 0.000000000000000000, 9.000000000000001776, 0.000000000000000000 ) ) ;
#10920=ORIENTED_EDGE ( 'NONE', *, *, #20472, .F. ) ;
#10922=CARTESIAN_POINT ( 'NONE',  ( 7.619520639128047002, 4.999999999999999112, 0.000000000000000000 ) ) ;
#10931=ORIENTED_EDGE ( 'NONE', *, *, #936, .F. ) ;
#10935=DIRECTION ( 'NONE',  ( 0.000000000000000000, 1.000000000000000000, 0.000000000000000000 ) ) ;
#10945=DIRECTION ( 'NONE',  ( 0.000000000000000000, 1.000000000000000000, -0.000000000000000000 ) ) ;
#10950=EDGE_CURVE ( 'NONE', #9451, #5395, #187, .T. ) ;
#10951=EDGE_LOOP ( 'NONE', ( #18471, #1769 ) ) ;
#10953=CARTESIAN_POINT ( 'NONE',  ( -18.98630159782011262, 9.000000000000001776, 1.000000000000000000 ) ) ;
#10958=CIRCLE ( 'NONE', #6273, 0.5000000000000000000 ) ;
#10965=CARTESIAN_POINT ( 'NONE',  ( 0.000000000000000000, 9.000000000000001776, 0.000000000000000000 ) ) ;
#10967=PLANE ( 'NONE',  #944 ) ;
#10972=ORIENTED_EDGE ( 'NONE', *, *, #6720, .F. ) ;
#10974=CARTESIAN_POINT ( 'NONE',  ( 20.00000000000000000, -5.999999999999994671, 2.000000000000000000 ) ) ;
#10979=ORIENTED_EDGE ( 'NONE', *, *, #12986, .T. ) ;
#10981=( NAMED_UNIT ( * ) PLANE_ANGLE_UNIT ( ) SI_UNIT ( $, .RADIAN. ) );
#10986=VERTEX_POINT ( 'NONE', #19546 ) ;
#10989=PLANE ( 'NONE',  #180 ) ;
#10998=CARTESIAN_POINT ( 'NONE',  ( 0.000000000000000000, 9.000000000000001776, 1.000000000000000000 ) ) ;
#11006=ORIENTED_EDGE ( 'NONE', *, *, #17304, .F. ) ;
#11011=ADVANCED_FACE ( 'NONE', ( #14607 ), #9907, .T. ) ;
#11013=AXIS2_PLACEMENT_3D ( 'NONE', #9081, #18499, #6534 ) ;
#11015=FACE_OUTER_BOUND ( 'NONE', #7045, .T. ) ;
#11017=DIRECTION ( 'NONE',  ( 1.000000000000000000, 0.000000000000000000, 0.000000000000000000 ) ) ;
#11019=EDGE_CURVE ( 'NONE', #7736, #8434, #16289, .T. ) ;
#11024=ORIENTED_EDGE ( 'NONE', *, *, #1690, .F. ) ;
#11032=DIRECTION ( 'NONE',  ( 1.000000000000000000, 0.000000000000000000, 0.000000000000000000 ) ) ;
#11033=CARTESIAN_POINT ( 'NONE',  ( 9.830951894845298966, -2.500000000000047518, 7.000000000000000000 ) ) ;
#11035=VECTOR ( 'NONE', #13265, 1000.000000000000000 ) ;
#11036=ORIENTED_EDGE ( 'NONE', *, *, #11983, .F. ) ;
#11037=DIRECTION ( 'NONE',  ( 1.000000000000000000, 0.000000000000000000, 0.000000000000000000 ) ) ;
#11046=CARTESIAN_POINT ( 'NONE',  ( 3.747260319564023501, 4.999999999999999112, 0.000000000000000000 ) ) ;
#11048=AXIS2_PLACEMENT_3D ( 'NONE', #3981, #18001, #747 ) ;
#11049=PLANE ( 'NONE',  #17993 ) ;
#11056=EDGE_LOOP ( 'NONE', ( #14328, #5601, #16034, #7768 ) ) ;
#11059=EDGE_LOOP ( 'NONE', ( #17097, #11772, #9356, #15473 ) ) ;
#11064=VECTOR ( 'NONE', #14243, 1000.000000000000000 ) ;
#11069=ORIENTED_EDGE ( 'NONE', *, *, #15911, .F. ) ;
#11076=CARTESIAN_POINT ( 'NONE',  ( -18.98630159782011262, 0.000000000000000000, 1.000000000000000000 ) ) ;
#11082=ORIENTED_EDGE ( 'NONE', *, *, #11845, .T. ) ;
#11085=ORIENTED_EDGE ( 'NONE', *, *, #15464, .F. ) ;
#11086=CARTESIAN_POINT ( 'NONE',  ( -0.1250000000000035805, 0.000000000000000000, 1.000000000000000000 ) ) ;
#11089=EDGE_CURVE ( 'NONE', #607, #19969, #8343, .T. ) ;
#11090=LINE ( 'NONE', #14206, #17144 ) ;
#11098=CARTESIAN_POINT ( 'NONE',  ( 6.183390479346035917, 0.000000000000000000, 1.000000000000000000 ) ) ;
#11102=EDGE_CURVE ( 'NONE', #9583, #1458, #6779, .T. ) ;
#11103=DIRECTION ( 'NONE',  ( -0.000000000000000000, -0.000000000000000000, -1.000000000000000000 ) ) ;
#11104=PLANE ( 'NONE',  #16092 ) ;
#11105=VECTOR ( 'NONE', #13337, 1000.000000000000000 ) ;
#11108=ORIENTED_EDGE ( 'NONE', *, *, #4167, .F. ) ;
#11111=ORIENTED_EDGE ( 'NONE', *, *, #17973, .F. ) ;
#11112=UNCERTAINTY_MEASURE_WITH_UNIT (LENGTH_MEASURE( 1.000000000000000082E-05 ), #4790, 'distance_accuracy_value', 'NONE');
#11118=VECTOR ( 'NONE', #2000, 1000.000000000000000 ) ;
#11128=EDGE_CURVE ( 'NONE', #8745, #10713, #11268, .T. ) ;
#11136=VECTOR ( 'NONE', #19895, 1000.000000000000000 ) ;
#11138=CARTESIAN_POINT ( 'NONE',  ( 0.000000000000000000, 9.000000000000001776, 0.000000000000000000 ) ) ;
#11145=DIRECTION ( 'NONE',  ( 0.000000000000000000, 0.000000000000000000, 1.000000000000000000 ) ) ;
#11148=DIRECTION ( 'NONE',  ( -0.000000000000000000, -0.000000000000000000, -1.000000000000000000 ) ) ;
#11154=EDGE_CURVE ( 'NONE', #6649, #19533, #19642, .T. ) ;
#11159=ORIENTED_EDGE ( 'NONE', *, *, #9585, .T. ) ;
#11162=ORIENTED_EDGE ( 'NONE', *, *, #8154, .F. ) ;
#11163=FACE_OUTER_BOUND ( 'NONE', #7630, .T. ) ;
#11164=ADVANCED_FACE ( 'NONE', ( #1760 ), #3322, .T. ) ;
#11166=ORIENTED_EDGE ( 'NONE', *, *, #3876, .F. ) ;
#11167=DIRECTION ( 'NONE',  ( 1.000000000000000000, 0.000000000000000000, 0.000000000000000000 ) ) ;
#11168=PLANE ( 'NONE',  #13636 ) ;
#11177=DIRECTION ( 'NONE',  ( -0.000000000000000000, -0.000000000000000000, -1.000000000000000000 ) ) ;
#11181=DIRECTION ( 'NONE',  ( 0.000000000000000000, 1.000000000000000000, 0.000000000000000000 ) ) ;
#11183=DIRECTION ( 'NONE',  ( 1.000000000000000000, 0.000000000000000000, 0.000000000000000000 ) ) ;
#11187=ORIENTED_EDGE ( 'NONE', *, *, #14623, .F. ) ;
#11197=EDGE_CURVE ( 'NONE', #5735, #1111, #20064, .T. ) ;
#11199=FACE_OUTER_BOUND ( 'NONE', #1509, .T. ) ;
#11202=AXIS2_PLACEMENT_3D ( 'NONE', #4295, #10790, #16943 ) ;
#11206=ORIENTED_EDGE ( 'NONE', *, *, #17229, .T. ) ;
#11211=CARTESIAN_POINT ( 'NONE',  ( 27.49999999999999645, -4.770489558936219510E-14, 0.000000000000000000 ) ) ;
#11216=CARTESIAN_POINT ( 'NONE',  ( -7.369520639128046113, 0.000000000000000000, 1.000000000000000000 ) ) ;
#11234=LINE ( 'NONE', #17725, #20484 ) ;
#11235=EDGE_CURVE ( 'NONE', #17247, #3944, #4251, .T. ) ;
#11237=CARTESIAN_POINT ( 'NONE',  ( 24.50000000000000000, 0.000000000000000000, 0.000000000000000000 ) ) ;
#11240=CARTESIAN_POINT ( 'NONE',  ( 15.36404127825609400, 9.000000000000001776, 1.000000000000000000 ) ) ;
#11241=FACE_OUTER_BOUND ( 'NONE', #8107, .T. ) ;
#11242=CARTESIAN_POINT ( 'NONE',  ( -27.52582389412042474, 4.853545418763153485, 1.000000000000000000 ) ) ;
#11254=VERTEX_POINT ( 'NONE', #807 ) ;
#11260=CARTESIAN_POINT ( 'NONE',  ( -1.561130159782011306, 4.999999999999999112, 1.000000000000000000 ) ) ;
#11268=LINE ( 'NONE', #2164, #19587 ) ;
#11272=DIRECTION ( 'NONE',  ( -1.000000000000000000, 0.000000000000000000, 0.000000000000000000 ) ) ;
#11274=ORIENTED_EDGE ( 'NONE', *, *, #5705, .T. ) ;
#11275=VECTOR ( 'NONE', #3135, 1000.000000000000000 ) ;
#11281=EDGE_LOOP ( 'NONE', ( #430, #8751, #11893, #12581 ) ) ;
#11285=CARTESIAN_POINT ( 'NONE',  ( 0.000000000000000000, 9.000000000000001776, 1.000000000000000000 ) ) ;
#11287=CARTESIAN_POINT ( 'NONE',  ( 0.000000000000000000, 9.000000000000001776, 0.000000000000000000 ) ) ;
#11297=EDGE_CURVE ( 'NONE', #7639, #4697, #6348, .T. ) ;
#11300=VECTOR ( 'NONE', #10765, 1000.000000000000000 ) ;
#11308=ORIENTED_EDGE ( 'NONE', *, *, #12509, .T. ) ;
#11328=VERTEX_POINT ( 'NONE', #12412 ) ;
#11333=DIRECTION ( 'NONE',  ( -0.000000000000000000, 0.000000000000000000, -1.000000000000000000 ) ) ;
#11335=VECTOR ( 'NONE', #8659, 1000.000000000000114 ) ;
#11336=ORIENTED_EDGE ( 'NONE', *, *, #1988, .F. ) ;
#11337=DIRECTION ( 'NONE',  ( -0.000000000000000000, -0.000000000000000000, -1.000000000000000000 ) ) ;
#11339=ORIENTED_EDGE ( 'NONE', *, *, #18283, .T. ) ;
#11344=LINE ( 'NONE', #14482, #3756 ) ;
#11360=CARTESIAN_POINT ( 'NONE',  ( 0.000000000000000000, 4.999999999999999112, 1.000000000000000000 ) ) ;
#11361=ORIENTED_EDGE ( 'NONE', *, *, #11546, .F. ) ;
#11362=DIRECTION ( 'NONE',  ( 0.000000000000000000, 0.000000000000000000, 1.000000000000000000 ) ) ;
#11364=ORIENTED_EDGE ( 'NONE', *, *, #4226, .F. ) ;
#11367=VECTOR ( 'NONE', #2105, 1000.000000000000000 ) ;
#11371=CARTESIAN_POINT ( 'NONE',  ( 15.36404127825609400, 0.000000000000000000, 0.000000000000000000 ) ) ;
#11375=ORIENTED_EDGE ( 'NONE', *, *, #11640, .F. ) ;
#11379=ORIENTED_EDGE ( 'NONE', *, *, #732, .F. ) ;
#11383=CARTESIAN_POINT ( 'NONE',  ( -17.11324865405191176, -11.00000000000000000, 2.000000000000000000 ) ) ;
#11405=EDGE_CURVE ( 'NONE', #17531, #19533, #14387, .T. ) ;
#11413=ORIENTED_EDGE ( 'NONE', *, *, #12162, .T. ) ;
#11415=ORIENTED_EDGE ( 'NONE', *, *, #17759, .T. ) ;
#11418=EDGE_CURVE ( 'NONE', #10336, #16327, #9379, .T. ) ;
#11423=LINE ( 'NONE', #7446, #10062 ) ;
#11433=EDGE_CURVE ( 'NONE', #19789, #4981, #9175, .T. ) ;
#11436=VERTEX_POINT ( 'NONE', #10953 ) ;
#11439=LINE ( 'NONE', #2023, #15014 ) ;
#11440=VECTOR ( 'NONE', #16425, 1000.000000000000000 ) ;
#11441=EDGE_LOOP ( 'NONE', ( #2273, #16789, #13742, #8277 ) ) ;
#11443=CARTESIAN_POINT ( 'NONE',  ( -9.805650798910056309, 0.000000000000000000, 1.000000000000000000 ) ) ;
#11445=LINE ( 'NONE', #6437, #20261 ) ;
#11446=DIRECTION ( 'NONE',  ( 0.000000000000000000, -0.000000000000000000, -1.000000000000000000 ) ) ;
#11452=PLANE ( 'NONE',  #10702 ) ;
#11454=DIRECTION ( 'NONE',  ( 1.000000000000000000, 0.000000000000000000, 0.000000000000000000 ) ) ;
#11456=VERTEX_POINT ( 'NONE', #8017 ) ;
#11462=VERTEX_POINT ( 'NONE', #15550 ) ;
#11465=LINE ( 'NONE', #8436, #6048 ) ;
#11467=ORIENTED_EDGE ( 'NONE', *, *, #1937, .F. ) ;
#11468=PLANE ( 'NONE',  #16743 ) ;
#11469=VERTEX_POINT ( 'NONE', #19120 ) ;
#11470=CARTESIAN_POINT ( 'NONE',  ( 9.555650798910054533, 0.000000000000000000, 1.000000000000000000 ) ) ;
#11471=VECTOR ( 'NONE', #1259, 1000.000000000000000 ) ;
#11475=EDGE_CURVE ( 'NONE', #16571, #19021, #4773, .T. ) ;
#11491=LINE ( 'NONE', #17870, #3987 ) ;
#11493=ORIENTED_EDGE ( 'NONE', *, *, #18347, .F. ) ;
#11498=EDGE_CURVE ( 'NONE', #19423, #14130, #6554, .T. ) ;
#11500=CARTESIAN_POINT ( 'NONE',  ( 19.73630159782011617, 0.000000000000000000, 1.000000000000000000 ) ) ;
#11508=DIRECTION ( 'NONE',  ( 1.000000000000000000, 0.000000000000000000, -0.000000000000000000 ) ) ;
#11516=VERTEX_POINT ( 'NONE', #3305 ) ;
#11517=LINE ( 'NONE', #13185, #11136 ) ;
#11521=CARTESIAN_POINT ( 'NONE',  ( 20.00000000000000000, -5.999999999999994671, 2.000000000000000000 ) ) ;
#11524=VECTOR ( 'NONE', #18578, 1000.000000000000000 ) ;
#11530=EDGE_CURVE ( 'NONE', #8356, #5395, #2149, .T. ) ;
#11531=ADVANCED_FACE ( 'NONE', ( #266 ), #16373, .T. ) ;
#11533=DIRECTION ( 'NONE',  ( 0.000000000000000000, 0.000000000000000000, 1.000000000000000000 ) ) ;
#11540=ORIENTED_EDGE ( 'NONE', *, *, #6925, .F. ) ;
#11543=AXIS2_PLACEMENT_3D ( 'NONE', #7875, #9337, #10913 ) ;
#11544=PLANE ( 'NONE',  #18252 ) ;
#11546=EDGE_CURVE ( 'NONE', #14385, #10351, #16059, .T. ) ;
#11547=CARTESIAN_POINT ( 'NONE',  ( -20.00000000000000000, 0.000000000000000000, 1.000000000000000000 ) ) ;
#11550=DIRECTION ( 'NONE',  ( 0.000000000000000000, 1.000000000000000000, 0.000000000000000000 ) ) ;
#11552=DIRECTION ( 'NONE',  ( -0.000000000000000000, -0.000000000000000000, -1.000000000000000000 ) ) ;
#11559=ORIENTED_EDGE ( 'NONE', *, *, #9741, .T. ) ;
#11562=VERTEX_POINT ( 'NONE', #2051 ) ;
#11566=ORIENTED_EDGE ( 'NONE', *, *, #5555, .T. ) ;
#11569=CARTESIAN_POINT ( 'NONE',  ( 0.000000000000000000, 9.000000000000001776, 1.000000000000000000 ) ) ;
#11576=EDGE_CURVE ( 'NONE', #7093, #10351, #11465, .T. ) ;
#11586=EDGE_CURVE ( 'NONE', #19129, #9899, #8227, .T. ) ;
#11587=CARTESIAN_POINT ( 'NONE',  ( 11.99178095869207006, 4.999999999999999112, 1.000000000000000000 ) ) ;
#11595=LINE ( 'NONE', #16409, #12611 ) ;
#11598=FACE_OUTER_BOUND ( 'NONE', #15931, .T. ) ;
#11623=LINE ( 'NONE', #3791, #2379 ) ;
#11625=VECTOR ( 'NONE', #18797, 1000.000000000000000 ) ;
#11634=EDGE_LOOP ( 'NONE', ( #13687, #8660, #6580, #10644 ) ) ;
#11635=EDGE_CURVE ( 'NONE', #4631, #16371, #14805, .T. ) ;
#11637=LINE ( 'NONE', #18028, #102 ) ;
#11638=DIRECTION ( 'NONE',  ( 1.000000000000000000, 0.000000000000000000, 0.000000000000000000 ) ) ;
#11640=EDGE_CURVE ( 'NONE', #4975, #11436, #19730, .T. ) ;
#11642=VECTOR ( 'NONE', #511, 1000.000000000000000 ) ;
#11647=DIRECTION ( 'NONE',  ( -1.000000000000000000, -0.000000000000000000, -0.000000000000000000 ) ) ;
#11648=DIRECTION ( 'NONE',  ( 0.000000000000000000, 0.000000000000000000, -1.000000000000000000 ) ) ;
#11660=ORIENTED_EDGE ( 'NONE', *, *, #8519, .T. ) ;
#11669=DIRECTION ( 'NONE',  ( 1.000000000000000000, 0.000000000000000000, 0.000000000000000000 ) ) ;
#11673=DIRECTION ( 'NONE',  ( 0.000000000000000000, 1.000000000000000000, 0.000000000000000000 ) ) ;
#11682=ORIENTED_EDGE ( 'NONE', *, *, #2751, .T. ) ;
#11685=DIRECTION ( 'NONE',  ( 1.000000000000000000, -0.000000000000000000, 0.000000000000000000 ) ) ;
#11697=VECTOR ( 'NONE', #18192, 1000.000000000000000 ) ;
#11701=AXIS2_PLACEMENT_3D ( 'NONE', #8912, #5979, #16951 ) ;
#11706=VECTOR ( 'NONE', #11854, 1000.000000000000000 ) ;
#11707=LINE ( 'NONE', #5441, #12615 ) ;
#11714=ORIENTED_EDGE ( 'NONE', *, *, #19303, .T. ) ;
#11718=ORIENTED_EDGE ( 'NONE', *, *, #2498, .T. ) ;
#11721=CARTESIAN_POINT ( 'NONE',  ( 0.000000000000000000, 4.999999999999999112, 1.000000000000000000 ) ) ;
#11725=VECTOR ( 'NONE', #13502, 1000.000000000000000 ) ;
#11727=FACE_OUTER_BOUND ( 'NONE', #12539, .T. ) ;
#11737=VECTOR ( 'NONE', #6945, 1000.000000000000000 ) ;
#11740=ORIENTED_EDGE ( 'NONE', *, *, #12802, .T. ) ;
#11746=FACE_OUTER_BOUND ( 'NONE', #10468, .T. ) ;
#11750=CARTESIAN_POINT ( 'NONE',  ( -21.42243175760212637, 4.999999999999999112, 1.000000000000000000 ) ) ;
#11759=ORIENTED_EDGE ( 'NONE', *, *, #11903, .F. ) ;
#11763=ORIENTED_EDGE ( 'NONE', *, *, #10270, .T. ) ;
#11769=FACE_OUTER_BOUND ( 'NONE', #7222, .T. ) ;
#11770=VERTEX_POINT ( 'NONE', #10201 ) ;
#11772=ORIENTED_EDGE ( 'NONE', *, *, #3366, .F. ) ;
#11773=PLANE ( 'NONE',  #10672 ) ;
#11775=CARTESIAN_POINT ( 'NONE',  ( -15.11404127825609223, 9.000000000000001776, 1.000000000000000000 ) ) ;
#11778=VECTOR ( 'NONE', #9747, 1000.000000000000000 ) ;
#11786=ORIENTED_EDGE ( 'NONE', *, *, #11433, .T. ) ;
#11787=EDGE_CURVE ( 'NONE', #7606, #8680, #2554, .T. ) ;
#11790=ORIENTED_EDGE ( 'NONE', *, *, #1913, .T. ) ;
#11793=CARTESIAN_POINT ( 'NONE',  ( 0.000000000000000000, -0.5000000000000004441, 0.5000000000000000000 ) ) ;
#11795=EDGE_LOOP ( 'NONE', ( #11036, #6985, #1892, #12827 ) ) ;
#11804=ADVANCED_FACE ( 'NONE', ( #15420 ), #3921, .F. ) ;
#11812=LINE ( 'NONE', #3659, #19100 ) ;
#11814=DIRECTION ( 'NONE',  ( -0.000000000000000000, 0.000000000000000000, -1.000000000000000000 ) ) ;
#11815=ORIENTED_EDGE ( 'NONE', *, *, #12092, .F. ) ;
#11816=ORIENTED_EDGE ( 'NONE', *, *, #17948, .T. ) ;
#11819=CARTESIAN_POINT ( 'NONE',  ( -5.933390479346035029, 9.000000000000001776, 0.000000000000000000 ) ) ;
#11823=DIRECTION ( 'NONE',  ( -0.000000000000000000, -0.000000000000000000, -1.000000000000000000 ) ) ;
#11824=CARTESIAN_POINT ( 'NONE',  ( 19.73630159782011617, 0.000000000000000000, 0.000000000000000000 ) ) ;
#11825=DIRECTION ( 'NONE',  ( -0.000000000000000000, 1.000000000000000000, -0.000000000000000000 ) ) ;
#11827=LINE ( 'NONE', #8806, #10200 ) ;
#11829=EDGE_CURVE ( 'NONE', #10647, #3720, #5492, .T. ) ;
#11834=DIRECTION ( 'NONE',  ( 0.000000000000000000, 1.000000000000000000, -0.000000000000000000 ) ) ;
#11844=ORIENTED_EDGE ( 'NONE', *, *, #5199, .F. ) ;
#11845=EDGE_CURVE ( 'NONE', #17, #17043, #20461, .T. ) ;
#11848=CARTESIAN_POINT ( 'NONE',  ( -15.11404127825609223, 9.000000000000001776, 1.000000000000000000 ) ) ;
#11853=CARTESIAN_POINT ( 'NONE',  ( 19.73630159782011617, 9.000000000000001776, 1.000000000000000000 ) ) ;
#11854=DIRECTION ( 'NONE',  ( -0.000000000000000000, -0.000000000000000000, -1.000000000000000000 ) ) ;
#11856=DIRECTION ( 'NONE',  ( 0.000000000000000000, 1.000000000000000000, 0.000000000000000000 ) ) ;
#11863=ORIENTED_EDGE ( 'NONE', *, *, #12533, .F. ) ;
#11866=CARTESIAN_POINT ( 'NONE',  ( 15.86404127825609400, 0.000000000000000000, 0.000000000000000000 ) ) ;
#11867=ORIENTED_EDGE ( 'NONE', *, *, #14265, .T. ) ;
#11870=ADVANCED_FACE ( 'NONE', ( #17292 ), #18780, .F. ) ;
#11876=CARTESIAN_POINT ( 'NONE',  ( -26.04469207716614321, -2.255140518769849223E-14, 1.000000000000000000 ) ) ;
#11881=FACE_OUTER_BOUND ( 'NONE', #10075, .T. ) ;
#11886=ORIENTED_EDGE ( 'NONE', *, *, #2254, .F. ) ;
#11889=VERTEX_POINT ( 'NONE', #18984 ) ;
#11890=CARTESIAN_POINT ( 'NONE',  ( -15.61404127825609223, 9.000000000000001776, 1.000000000000000000 ) ) ;
#11891=CARTESIAN_POINT ( 'NONE',  ( 20.00000000000000000, -5.999999999999994671, 2.000000000000000000 ) ) ;
#11893=ORIENTED_EDGE ( 'NONE', *, *, #12459, .T. ) ;
#11895=EDGE_CURVE ( 'NONE', #13440, #5494, #4640, .T. ) ;
#11897=FACE_OUTER_BOUND ( 'NONE', #19481, .T. ) ;
#11902=DIRECTION ( 'NONE',  ( -0.000000000000000000, -0.000000000000000000, -1.000000000000000000 ) ) ;
#11903=EDGE_CURVE ( 'NONE', #19625, #18278, #5905, .T. ) ;
#11904=CARTESIAN_POINT ( 'NONE',  ( 0.000000000000000000, 9.000000000000001776, 1.000000000000000000 ) ) ;
#11905=DIRECTION ( 'NONE',  ( -0.000000000000000000, -0.000000000000000000, -1.000000000000000000 ) ) ;
#11914=DIRECTION ( 'NONE',  ( 1.000000000000000000, 0.000000000000000000, 0.000000000000000000 ) ) ;
#11916=ORIENTED_EDGE ( 'NONE', *, *, #13115, .F. ) ;
#11921=ADVANCED_FACE ( 'NONE', ( #20247 ), #3182, .T. ) ;
#11923=AXIS2_PLACEMENT_3D ( 'NONE', #18841, #20106, #13804 ) ;
#11924=PLANE ( 'NONE',  #11048 ) ;
#11925=DIRECTION ( 'NONE',  ( 0.000000000000000000, -0.000000000000000000, 1.000000000000000000 ) ) ;
#11934=EDGE_CURVE ( 'NONE', #19548, #13158, #9351, .T. ) ;
#11939=ORIENTED_EDGE ( 'NONE', *, *, #3383, .T. ) ;
#11942=CARTESIAN_POINT ( 'NONE',  ( -5.933390479346035029, 0.000000000000000000, 1.000000000000000000 ) ) ;
#11945=EDGE_LOOP ( 'NONE', ( #16782, #14512, #9327, #8459 ) ) ;
#11946=EDGE_CURVE ( 'NONE', #510, #15982, #2872, .T. ) ;
#11948=DIRECTION ( 'NONE',  ( 1.000000000000000000, 0.000000000000000000, 0.000000000000000000 ) ) ;
#11965=VERTEX_POINT ( 'NONE', #9249 ) ;
#11968=ORIENTED_EDGE ( 'NONE', *, *, #19488, .T. ) ;
#11970=LINE ( 'NONE', #10515, #13703 ) ;
#11971=AXIS2_PLACEMENT_3D ( 'NONE', #13392, #16626, #15268 ) ;
#11972=ORIENTED_EDGE ( 'NONE', *, *, #9611, .F. ) ;
#11975=VERTEX_POINT ( 'NONE', #5924 ) ;
#11976=DIRECTION ( 'NONE',  ( -0.000000000000000000, -0.000000000000000000, -1.000000000000000000 ) ) ;
#11979=AXIS2_PLACEMENT_3D ( 'NONE', #8541, #14912, #7083 ) ;
#11983=EDGE_CURVE ( 'NONE', #4521, #9180, #12295, .T. ) ;
#11989=DIRECTION ( 'NONE',  ( -0.000000000000000000, -0.000000000000000000, -1.000000000000000000 ) ) ;
#11998=EDGE_LOOP ( 'NONE', ( #14928, #19431, #15874, #9603 ) ) ;
#11999=CIRCLE ( 'NONE', #12665, 0.4999999999999987232 ) ;
#12000=AXIS2_PLACEMENT_3D ( 'NONE', #11876, #2563, #12088 ) ;
#12003=AXIS2_PLACEMENT_3D ( 'NONE', #12361, #14225, #6289 ) ;
#12015=ORIENTED_EDGE ( 'NONE', *, *, #19901, .T. ) ;
#12025=PLANE ( 'NONE',  #18496 ) ;
#12028=VECTOR ( 'NONE', #15248, 1000.000000000000000 ) ;
#12029=LINE ( 'NONE', #5659, #2025 ) ;
#12030=DIRECTION ( 'NONE',  ( 1.000000000000000000, 0.000000000000000000, 0.000000000000000000 ) ) ;
#12031=CARTESIAN_POINT ( 'NONE',  ( 0.000000000000000000, 9.000000000000001776, 1.000000000000000000 ) ) ;
#12032=VECTOR ( 'NONE', #2811, 1000.000000000000000 ) ;
#12039=PLANE ( 'NONE',  #17645 ) ;
#12040=CARTESIAN_POINT ( 'NONE',  ( -19.48630159782011262, 4.999999999999999112, 0.000000000000000000 ) ) ;
#12042=EDGE_CURVE ( 'NONE', #17483, #16676, #14072, .T. ) ;
#12043=DIRECTION ( 'NONE',  ( -0.000000000000000000, -0.000000000000000000, -1.000000000000000000 ) ) ;
#12049=EDGE_CURVE ( 'NONE', #19600, #7153, #4148, .T. ) ;
#12051=ADVANCED_FACE ( 'NONE', ( #18487 ), #7598, .F. ) ;
#12053=VECTOR ( 'NONE', #14902, 1000.000000000000000 ) ;
#12056=VECTOR ( 'NONE', #15914, 1000.000000000000000 ) ;
#12057=VERTEX_POINT ( 'NONE', #9168 ) ;
#12058=CARTESIAN_POINT ( 'NONE',  ( -7.869520639128047002, 9.000000000000001776, 1.000000000000000000 ) ) ;
#12062=LINE ( 'NONE', #4323, #6663 ) ;
#12064=CARTESIAN_POINT ( 'NONE',  ( 0.000000000000000000, 9.000000000000001776, 1.000000000000000000 ) ) ;
#12067=EDGE_CURVE ( 'NONE', #4874, #1688, #15541, .T. ) ;
#12076=ORIENTED_EDGE ( 'NONE', *, *, #796, .T. ) ;
#12084=ADVANCED_FACE ( 'NONE', ( #12194 ), #20062, .T. ) ;
#12086=ORIENTED_EDGE ( 'NONE', *, *, #12158, .T. ) ;
#12088=DIRECTION ( 'NONE',  ( -8.673617379884033500E-16, 1.000000000000000000, 0.000000000000000000 ) ) ;
#12089=DIRECTION ( 'NONE',  ( 0.000000000000000000, 0.000000000000000000, 1.000000000000000000 ) ) ;
#12091=CARTESIAN_POINT ( 'NONE',  ( -14.00000000000000000, 0.000000000000000000, 1.000000000000000000 ) ) ;
#12092=EDGE_CURVE ( 'NONE', #19648, #15034, #1125, .T. ) ;
#12101=VECTOR ( 'NONE', #5287, 1000.000000000000000 ) ;
#12106=ORIENTED_EDGE ( 'NONE', *, *, #13242, .T. ) ;
#12107=DIRECTION ( 'NONE',  ( -1.000000000000000000, 0.000000000000000000, 0.000000000000000000 ) ) ;
#12109=ORIENTED_EDGE ( 'NONE', *, *, #19139, .T. ) ;
#12115=DIRECTION ( 'NONE',  ( 0.000000000000000000, 0.000000000000000000, 1.000000000000000000 ) ) ;
#12125=DIRECTION ( 'NONE',  ( -0.000000000000000000, -0.000000000000000000, -1.000000000000000000 ) ) ;
#12130=ORIENTED_EDGE ( 'NONE', *, *, #661, .T. ) ;
#12133=LINE ( 'NONE', #18731, #2783 ) ;
#12136=CARTESIAN_POINT ( 'NONE',  ( 15.86404127825609400, 9.000000000000001776, 1.000000000000000000 ) ) ;
#12139=DIRECTION ( 'NONE',  ( 0.000000000000000000, -0.000000000000000000, 1.000000000000000000 ) ) ;
#12143=DIRECTION ( 'NONE',  ( -1.000000000000000000, 0.000000000000000000, 0.000000000000000000 ) ) ;
#12145=DIRECTION ( 'NONE',  ( -0.000000000000000000, 0.000000000000000000, -1.000000000000000000 ) ) ;
#12157=PLANE ( 'NONE',  #6103 ) ;
#12158=EDGE_CURVE ( 'NONE', #11516, #2248, #18902, .T. ) ;
#12162=EDGE_CURVE ( 'NONE', #19, #14460, #2996, .T. ) ;
#12164=PLANE ( 'NONE',  #10203 ) ;
#12165=LINE ( 'NONE', #5690, #13491 ) ;
#12167=CARTESIAN_POINT ( 'NONE',  ( 25.04469207716615031, 9.000000000000001776, 0.000000000000000000 ) ) ;
#12176=VERTEX_POINT ( 'NONE', #10531 ) ;
#12194=FACE_OUTER_BOUND ( 'NONE', #3391, .T. ) ;
#12195=VECTOR ( 'NONE', #9949, 1000.000000000000000 ) ;
#12196=VECTOR ( 'NONE', #16195, 1000.000000000000000 ) ;
#12198=CARTESIAN_POINT ( 'NONE',  ( -25.29469207716615031, 4.999999999999999112, 1.000000000000000000 ) ) ;
#12211=EDGE_CURVE ( 'NONE', #8663, #3716, #9372, .T. ) ;
#12214=DIRECTION ( 'NONE',  ( 0.000000000000000000, 1.000000000000000000, 0.000000000000000000 ) ) ;
#12217=FACE_OUTER_BOUND ( 'NONE', #12718, .T. ) ;
#12224=EDGE_LOOP ( 'NONE', ( #5881, #11467, #9278, #14575 ) ) ;
#12229=CARTESIAN_POINT ( 'NONE',  ( -20.92243175760212637, 4.999999999999999112, 0.000000000000000000 ) ) ;
#12230=VERTEX_POINT ( 'NONE', #9677 ) ;
#12233=DIRECTION ( 'NONE',  ( 1.000000000000000000, 0.000000000000000000, 0.000000000000000000 ) ) ;
#12234=ORIENTED_EDGE ( 'NONE', *, *, #19862, .T. ) ;
#12238=CARTESIAN_POINT ( 'NONE',  ( 5.683390479346035029, 9.000000000000001776, 1.000000000000000000 ) ) ;
#12241=AXIS2_PLACEMENT_3D ( 'NONE', #16255, #9562, #153 ) ;
#12251=VERTEX_POINT ( 'NONE', #10268 ) ;
#12254=EDGE_LOOP ( 'NONE', ( #7280, #19300, #908, #5446 ) ) ;
#12256=DIRECTION ( 'NONE',  ( 0.000000000000000000, -1.000000000000000000, 0.000000000000000000 ) ) ;
#12261=DIRECTION ( 'NONE',  ( 0.000000000000000000, -0.000000000000000000, 1.000000000000000000 ) ) ;
#12262=LINE ( 'NONE', #9137, #9203 ) ;
#12271=EDGE_CURVE ( 'NONE', #4847, #9411, #3577, .T. ) ;
#12278=ORIENTED_EDGE ( 'NONE', *, *, #17722, .T. ) ;
#12279=ORIENTED_EDGE ( 'NONE', *, *, #7427, .T. ) ;
#12285=CARTESIAN_POINT ( 'NONE',  ( -5.933390479346035029, 9.000000000000001776, 1.000000000000000000 ) ) ;
#12295=LINE ( 'NONE', #2891, #10039 ) ;
#12299=EDGE_CURVE ( 'NONE', #9021, #4521, #759, .T. ) ;
#12302=ORIENTED_EDGE ( 'NONE', *, *, #970, .T. ) ;
#12306=DIRECTION ( 'NONE',  ( 1.000000000000000000, 0.000000000000000000, 0.000000000000000000 ) ) ;
#12309=EDGE_CURVE ( 'NONE', #16469, #13516, #10583, .T. ) ;
#12310=EDGE_CURVE ( 'NONE', #14610, #8663, #5038, .T. ) ;
#12324=EDGE_CURVE ( 'NONE', #2944, #4223, #10483, .T. ) ;
#12330=CARTESIAN_POINT ( 'NONE',  ( 11.49178095869207006, 4.999999999999999112, 1.000000000000000000 ) ) ;
#12331=AXIS2_PLACEMENT_3D ( 'NONE', #6684, #11181, #17657 ) ;
#12337=SURFACE_STYLE_FILL_AREA ( #1260 ) ;
#12339=LINE ( 'NONE', #10572, #770 ) ;
#12341=ADVANCED_FACE ( 'NONE', ( #2740 ), #10377, .T. ) ;
#12343=FACE_OUTER_BOUND ( 'NONE', #15466, .T. ) ;
#12344=DIRECTION ( 'NONE',  ( 0.000000000000000000, 0.000000000000000000, 1.000000000000000000 ) ) ;
#12347=DIRECTION ( 'NONE',  ( 1.000000000000000000, 0.000000000000000000, 0.000000000000000000 ) ) ;
#12351=VECTOR ( 'NONE', #14121, 1000.000000000000000 ) ;
#12352=ADVANCED_FACE ( 'NONE', ( #12354 ), #2520, .T. ) ;
#12353=ADVANCED_FACE ( 'NONE', ( #7144 ), #15280, .T. ) ;
#12354=FACE_OUTER_BOUND ( 'NONE', #15425, .T. ) ;
#12360=VECTOR ( 'NONE', #7780, 1000.000000000000000 ) ;
#12361=CARTESIAN_POINT ( 'NONE',  ( -0.1250000000000035805, 0.000000000000000000, 1.000000000000000000 ) ) ;
#12363=ORIENTED_EDGE ( 'NONE', *, *, #17788, .F. ) ;
#12372=CARTESIAN_POINT ( 'NONE',  ( 0.000000000000000000, 4.999999999999999112, 1.000000000000000000 ) ) ;
#12373=LINE ( 'NONE', #4434, #16079 ) ;
#12375=PLANE ( 'NONE',  #3627 ) ;
#12378=ORIENTED_EDGE ( 'NONE', *, *, #9847, .T. ) ;
#12382=VECTOR ( 'NONE', #17497, 1000.000000000000000 ) ;
#12387=ORIENTED_EDGE ( 'NONE', *, *, #3665, .T. ) ;
#12388=ORIENTED_EDGE ( 'NONE', *, *, #7331, .F. ) ;
#12396=VECTOR ( 'NONE', #14347, 1000.000000000000000 ) ;
#12401=CARTESIAN_POINT ( 'NONE',  ( 0.000000000000000000, 0.000000000000000000, 0.5000000000000000000 ) ) ;
#12402=DIRECTION ( 'NONE',  ( 0.000000000000000000, -0.000000000000000000, 1.000000000000000000 ) ) ;
#12412=CARTESIAN_POINT ( 'NONE',  ( -17.05017143803810242, 4.999999999999999112, 1.000000000000000000 ) ) ;
#12418=ORIENTED_EDGE ( 'NONE', *, *, #13111, .F. ) ;
#12419=CARTESIAN_POINT ( 'NONE',  ( 0.000000000000000000, 4.999999999999999112, 1.000000000000000000 ) ) ;
#12420=CARTESIAN_POINT ( 'NONE',  ( 0.000000000000000000, 4.999999999999999112, 1.000000000000000000 ) ) ;
#12424=CARTESIAN_POINT ( 'NONE',  ( 13.92791111847407848, 4.999999999999999112, 1.000000000000000000 ) ) ;
#12428=EDGE_CURVE ( 'NONE', #1844, #1315, #20008, .T. ) ;
#12435=VERTEX_POINT ( 'NONE', #1171 ) ;
#12442=SURFACE_STYLE_USAGE ( .BOTH. , #20412 ) ;
#12444=AXIS2_PLACEMENT_3D ( 'NONE', #2027, #3804, #2227 ) ;
#12446=ORIENTED_EDGE ( 'NONE', *, *, #16038, .T. ) ;
#12448=PLANE ( 'NONE',  #11923 ) ;
#12457=CARTESIAN_POINT ( 'NONE',  ( -23.35856191738413656, 0.000000000000000000, 0.000000000000000000 ) ) ;
#12459=EDGE_CURVE ( 'NONE', #9247, #19171, #20315, .T. ) ;
#12465=ORIENTED_EDGE ( 'NONE', *, *, #6734, .T. ) ;
#12466=ORIENTED_EDGE ( 'NONE', *, *, #17229, .F. ) ;
#12470=EDGE_CURVE ( 'NONE', #17893, #9631, #7949, .T. ) ;
#12474=CARTESIAN_POINT ( 'NONE',  ( 27.52582389412042474, 4.853545418763153485, 1.000000000000000000 ) ) ;
#12475=LINE ( 'NONE', #2858, #7537 ) ;
#12476=CARTESIAN_POINT ( 'NONE',  ( -23.35856191738413656, 9.000000000000001776, 1.000000000000000000 ) ) ;
#12477=CARTESIAN_POINT ( 'NONE',  ( 23.60856191738414012, 9.000000000000001776, 1.000000000000000000 ) ) ;
#12483=CARTESIAN_POINT ( 'NONE',  ( 17.80017143803810242, 9.000000000000001776, 0.000000000000000000 ) ) ;
#12484=EDGE_CURVE ( 'NONE', #15255, #8718, #6184, .T. ) ;
#12499=DIRECTION ( 'NONE',  ( 0.000000000000000000, -0.000000000000000000, 1.000000000000000000 ) ) ;
#12509=EDGE_CURVE ( 'NONE', #10573, #19423, #4820, .T. ) ;
#12513=DIRECTION ( 'NONE',  ( 0.000000000000000000, -1.000000000000000000, 0.000000000000000000 ) ) ;
#12518=VECTOR ( 'NONE', #20574, 1000.000000000000000 ) ;
#12521=CARTESIAN_POINT ( 'NONE',  ( -15.61404127825609223, 0.000000000000000000, 1.000000000000000000 ) ) ;
#12531=CARTESIAN_POINT ( 'NONE',  ( -11.74178095869206828, 4.999999999999999112, 1.000000000000000000 ) ) ;
#12533=EDGE_CURVE ( 'NONE', #4449, #15703, #7651, .T. ) ;
#12535=DIRECTION ( 'NONE',  ( -0.000000000000000000, -0.000000000000000000, -1.000000000000000000 ) ) ;
#12536=ORIENTED_EDGE ( 'NONE', *, *, #10784, .T. ) ;
#12537=CARTESIAN_POINT ( 'NONE',  ( -13.67791111847408025, 0.000000000000000000, 1.000000000000000000 ) ) ;
#12539=EDGE_LOOP ( 'NONE', ( #4445, #10831, #12302, #9843 ) ) ;
#12541=ADVANCED_FACE ( 'NONE', ( #17682 ), #6396, .T. ) ;
#12545=PLANE ( 'NONE',  #2843 ) ;
#12547=LINE ( 'NONE', #17362, #15696 ) ;
#12551=DIRECTION ( 'NONE',  ( 1.000000000000000000, 0.000000000000000000, 0.000000000000000000 ) ) ;
#12553=EDGE_CURVE ( 'NONE', #2453, #12804, #115, .T. ) ;
#12556=ORIENTED_EDGE ( 'NONE', *, *, #4892, .F. ) ;
#12562=ORIENTED_EDGE ( 'NONE', *, *, #14847, .F. ) ;
#12578=EDGE_CURVE ( 'NONE', #20304, #5740, #4714, .T. ) ;
#12581=ORIENTED_EDGE ( 'NONE', *, *, #12919, .T. ) ;
#12584=CARTESIAN_POINT ( 'NONE',  ( 6.183390479346035917, 4.999999999999999112, 1.000000000000000000 ) ) ;
#12585=DIRECTION ( 'NONE',  ( 0.000000000000000000, 1.000000000000000000, 0.000000000000000000 ) ) ;
#12586=ORIENTED_EDGE ( 'NONE', *, *, #5615, .F. ) ;
#12588=LINE ( 'NONE', #4751, #19794 ) ;
#12589=VECTOR ( 'NONE', #5653, 1000.000000000000000 ) ;
#12590=CARTESIAN_POINT ( 'NONE',  ( -5.999999999999999112, -7.500000000000047073, 8.999999999999998224 ) ) ;
#12593=ADVANCED_FACE ( 'NONE', ( #11199 ), #12861, .F. ) ;
#12598=PLANE ( 'NONE',  #2410 ) ;
#12600=CARTESIAN_POINT ( 'NONE',  ( 26.04469207716615031, 9.000000000000001776, 1.000000000000000000 ) ) ;
#12611=VECTOR ( 'NONE', #2085, 1000.000000000000000 ) ;
#12615=VECTOR ( 'NONE', #19367, 1000.000000000000000 ) ;
#12618=EDGE_CURVE ( 'NONE', #9549, #15974, #17367, .T. ) ;
#12621=CARTESIAN_POINT ( 'NONE',  ( 2.311130159782011972, 9.000000000000001776, 0.000000000000000000 ) ) ;
#12624=CARTESIAN_POINT ( 'NONE',  ( 7.619520639128047002, 0.000000000000000000, 0.000000000000000000 ) ) ;
#12634=LINE ( 'NONE', #17147, #12653 ) ;
#12637=ORIENTED_EDGE ( 'NONE', *, *, #19226, .F. ) ;
#12639=DIRECTION ( 'NONE',  ( 0.1736481776669295263, -0.9848077530122082424, 0.000000000000000000 ) ) ;
#12643=LINE ( 'NONE', #14116, #17632 ) ;
#12653=VECTOR ( 'NONE', #17243, 1000.000000000000000 ) ;
#12660=PLANE ( 'NONE',  #656 ) ;
#12662=VERTEX_POINT ( 'NONE', #19166 ) ;
#12664=VECTOR ( 'NONE', #5097, 1000.000000000000000 ) ;
#12665=AXIS2_PLACEMENT_3D ( 'NONE', #15740, #12089, #18481 ) ;
#12674=DIRECTION ( 'NONE',  ( -0.000000000000000000, -0.000000000000000000, -1.000000000000000000 ) ) ;
#12679=EDGE_CURVE ( 'NONE', #9180, #6959, #8376, .T. ) ;
#12680=ORIENTED_EDGE ( 'NONE', *, *, #15015, .F. ) ;
#12690=DIRECTION ( 'NONE',  ( -0.000000000000000000, -0.000000000000000000, -1.000000000000000000 ) ) ;
#12691=CARTESIAN_POINT ( 'NONE',  ( -22.85856191738413656, 9.000000000000001776, 0.000000000000000000 ) ) ;
#12696=DIRECTION ( 'NONE',  ( -0.000000000000000000, 0.000000000000000000, -1.000000000000000000 ) ) ;
#12697=VECTOR ( 'NONE', #19542, 1000.000000000000000 ) ;
#12705=VECTOR ( 'NONE', #2794, 1000.000000000000000 ) ;
#12707=CARTESIAN_POINT ( 'NONE',  ( 0.3749999999999968914, 0.000000000000000000, 1.000000000000000000 ) ) ;
#12708=CARTESIAN_POINT ( 'NONE',  ( 2.311130159782011972, 4.999999999999999112, 1.000000000000000000 ) ) ;
#12709=LINE ( 'NONE', #13018, #6389 ) ;
#12715=ORIENTED_EDGE ( 'NONE', *, *, #17145, .T. ) ;
#12718=EDGE_LOOP ( 'NONE', ( #8258, #10273, #406, #19290, #7983, #1909, #16522, #6910, #13464, #12106 ) ) ;
#12721=ORIENTED_EDGE ( 'NONE', *, *, #17948, .F. ) ;
#12722=LINE ( 'NONE', #19125, #20131 ) ;
#12723=AXIS2_PLACEMENT_3D ( 'NONE', #6804, #11508, #13380 ) ;
#12725=AXIS2_PLACEMENT_3D ( 'NONE', #11098, #19160, #17676 ) ;
#12729=ADVANCED_FACE ( 'NONE', ( #622 ), #16219, .T. ) ;
#12732=CARTESIAN_POINT ( 'NONE',  ( 0.000000000000000000, 9.000000000000001776, 0.000000000000000000 ) ) ;
#12738=ORIENTED_EDGE ( 'NONE', *, *, #15346, .T. ) ;
#12740=CARTESIAN_POINT ( 'NONE',  ( 25.04469207716615031, 0.000000000000000000, 1.000000000000000000 ) ) ;
#12744=CARTESIAN_POINT ( 'NONE',  ( 21.17243175760212637, 4.999999999999999112, 1.000000000000000000 ) ) ;
#12748=ORIENTED_EDGE ( 'NONE', *, *, #8976, .F. ) ;
#12768=ORIENTED_EDGE ( 'NONE', *, *, #15152, .F. ) ;
#12774=CARTESIAN_POINT ( 'NONE',  ( -20.92243175760212637, 0.000000000000000000, 1.000000000000000000 ) ) ;
#12776=EDGE_CURVE ( 'NONE', #8019, #15255, #16315, .T. ) ;
#12782=CARTESIAN_POINT ( 'NONE',  ( 4.247260319564023945, 9.000000000000001776, 1.000000000000000000 ) ) ;
#12783=FACE_OUTER_BOUND ( 'NONE', #18024, .T. ) ;
#12786=ORIENTED_EDGE ( 'NONE', *, *, #6571, .F. ) ;
#12790=AXIS2_PLACEMENT_3D ( 'NONE', #9612, #15995, #16108 ) ;
#12796=ORIENTED_EDGE ( 'NONE', *, *, #20280, .F. ) ;
#12801=DIRECTION ( 'NONE',  ( 1.000000000000000000, 0.000000000000000000, -0.000000000000000000 ) ) ;
#12802=EDGE_CURVE ( 'NONE', #4223, #13134, #11812, .T. ) ;
#12804=VERTEX_POINT ( 'NONE', #5333 ) ;
#12808=FACE_OUTER_BOUND ( 'NONE', #11795, .T. ) ;
#12811=DIRECTION ( 'NONE',  ( 0.000000000000000000, -1.000000000000000000, 0.000000000000000000 ) ) ;
#12812=LINE ( 'NONE', #17837, #5368 ) ;
#12818=EDGE_LOOP ( 'NONE', ( #16706, #6576, #19555, #6531 ) ) ;
#12820=CARTESIAN_POINT ( 'NONE',  ( -26.79469207716615387, 9.000000000000001776, 1.000000000000000000 ) ) ;
#12821=EDGE_LOOP ( 'NONE', ( #17529, #35, #4309, #99 ) ) ;
#12827=ORIENTED_EDGE ( 'NONE', *, *, #2628, .T. ) ;
#12833=CARTESIAN_POINT ( 'NONE',  ( 0.000000000000000000, 4.999999999999999112, 1.000000000000000000 ) ) ;
#12841=ORIENTED_EDGE ( 'NONE', *, *, #959, .F. ) ;
#12843=EDGE_CURVE ( 'NONE', #8244, #42, #11707, .T. ) ;
#12851=VERTEX_POINT ( 'NONE', #15467 ) ;
#12853=PLANE ( 'NONE',  #4925 ) ;
#12861=PLANE ( 'NONE',  #10730 ) ;
#12869=ORIENTED_EDGE ( 'NONE', *, *, #16436, .F. ) ;
#12873=VERTEX_POINT ( 'NONE', #7118 ) ;
#12875=LINE ( 'NONE', #17380, #15455 ) ;
#12877=DIRECTION ( 'NONE',  ( 0.000000000000000000, 1.000000000000000000, 0.000000000000000000 ) ) ;
#12880=ADVANCED_FACE ( 'NONE', ( #13891 ), #10243, .F. ) ;
#12884=DIRECTION ( 'NONE',  ( 0.000000000000000000, 1.000000000000000000, 0.000000000000000000 ) ) ;
#12887=EDGE_LOOP ( 'NONE', ( #6292, #845, #8524, #18287, #12796, #20348, #7539, #5759, #3664, #14153 ) ) ;
#12889=FACE_OUTER_BOUND ( 'NONE', #17124, .T. ) ;
#12892=VERTEX_POINT ( 'NONE', #10461 ) ;
#12897=VERTEX_POINT ( 'NONE', #19884 ) ;
#12898=DIRECTION ( 'NONE',  ( -0.000000000000000000, -0.000000000000000000, -1.000000000000000000 ) ) ;
#12907=CARTESIAN_POINT ( 'NONE',  ( 5.999999999999999112, -7.500000000000047073, 8.999999999999998224 ) ) ;
#12908=FACE_OUTER_BOUND ( 'NONE', #16915, .T. ) ;
#12909=DIRECTION ( 'NONE',  ( 0.000000000000000000, 1.000000000000000000, -0.000000000000000000 ) ) ;
#12919=EDGE_CURVE ( 'NONE', #19171, #6959, #5754, .T. ) ;
#12932=LINE ( 'NONE', #19335, #2279 ) ;
#12942=EDGE_CURVE ( 'NONE', #5157, #7736, #19038, .T. ) ;
#12948=VERTEX_POINT ( 'NONE', #4588 ) ;
#12953=LINE ( 'NONE', #7847, #20317 ) ;
#12955=LINE ( 'NONE', #11287, #16812 ) ;
#12969=VECTOR ( 'NONE', #18385, 1000.000000000000000 ) ;
#12978=DIRECTION ( 'NONE',  ( -0.000000000000000000, 0.000000000000000000, -1.000000000000000000 ) ) ;
#12981=VECTOR ( 'NONE', #6840, 1000.000000000000000 ) ;
#12985=VECTOR ( 'NONE', #2206, 1000.000000000000000 ) ;
#12986=EDGE_CURVE ( 'NONE', #12435, #3029, #10225, .T. ) ;
#12995=CARTESIAN_POINT ( 'NONE',  ( 0.000000000000000000, 4.999999999999999112, 0.000000000000000000 ) ) ;
#13005=EDGE_CURVE ( 'NONE', #1137, #7916, #5208, .T. ) ;
#13008=LINE ( 'NONE', #4853, #1758 ) ;
#13015=LINE ( 'NONE', #9674, #1345 ) ;
#13018=CARTESIAN_POINT ( 'NONE',  ( -0.1250000000000035805, 9.000000000000000000, 1.000000000000000000 ) ) ;
#13023=VECTOR ( 'NONE', #20190, 1000.000000000000000 ) ;
#13025=ORIENTED_EDGE ( 'NONE', *, *, #11102, .F. ) ;
#13027=CARTESIAN_POINT ( 'NONE',  ( 9.555650798910054533, 4.999999999999999112, 1.000000000000000000 ) ) ;
#13036=ORIENTED_EDGE ( 'NONE', *, *, #4649, .F. ) ;
#13039=AXIS2_PLACEMENT_3D ( 'NONE', #8184, #6817, #4931 ) ;
#13051=ORIENTED_EDGE ( 'NONE', *, *, #6918, .F. ) ;
#13053=VECTOR ( 'NONE', #10716, 1000.000000000000000 ) ;
#13066=EDGE_CURVE ( 'NONE', #10351, #8244, #10958, .T. ) ;
#13069=FACE_OUTER_BOUND ( 'NONE', #12887, .T. ) ;
#13078=ORIENTED_EDGE ( 'NONE', *, *, #2847, .F. ) ;
#13079=ORIENTED_EDGE ( 'NONE', *, *, #7565, .T. ) ;
#13085=EDGE_CURVE ( 'NONE', #5367, #5490, #9816, .T. ) ;
#13100=DIRECTION ( 'NONE',  ( -1.000000000000000000, 0.000000000000000000, 0.000000000000000000 ) ) ;
#13107=VECTOR ( 'NONE', #8077, 1000.000000000000000 ) ;
#13109=ADVANCED_FACE ( 'NONE', ( #5418 ), #8555, .T. ) ;
#13110=ORIENTED_EDGE ( 'NONE', *, *, #15990, .T. ) ;
#13111=EDGE_CURVE ( 'NONE', #14385, #9688, #1867, .T. ) ;
#13112=LINE ( 'NONE', #17921, #17128 ) ;
#13114=CARTESIAN_POINT ( 'NONE',  ( 0.000000000000000000, 4.999999999999999112, 0.000000000000000000 ) ) ;
#13115=EDGE_CURVE ( 'NONE', #7202, #12948, #5110, .T. ) ;
#13117=LINE ( 'NONE', #10086, #3654 ) ;
#13123=PLANE ( 'NONE',  #956 ) ;
#13131=ORIENTED_EDGE ( 'NONE', *, *, #19227, .F. ) ;
#13134=VERTEX_POINT ( 'NONE', #13252 ) ;
#13137=ORIENTED_EDGE ( 'NONE', *, *, #7884, .F. ) ;
#13138=DIRECTION ( 'NONE',  ( 1.000000000000000000, 0.000000000000000000, 0.000000000000000000 ) ) ;
#13142=CARTESIAN_POINT ( 'NONE',  ( 25.54469207716615031, 4.999999999999999112, 1.000000000000000000 ) ) ;
#13149=CARTESIAN_POINT ( 'NONE',  ( -15.11404127825609223, 0.000000000000000000, 1.000000000000000000 ) ) ;
#13155=ORIENTED_EDGE ( 'NONE', *, *, #7079, .F. ) ;
#13156=CARTESIAN_POINT ( 'NONE',  ( 27.49999999999999645, -4.770489558936219510E-14, 1.000000000000000000 ) ) ;
#13158=VERTEX_POINT ( 'NONE', #294 ) ;
#13160=ORIENTED_EDGE ( 'NONE', *, *, #19492, .F. ) ;
#13162=EDGE_LOOP ( 'NONE', ( #6738, #8054, #11159, #12738 ) ) ;
#13167=CARTESIAN_POINT ( 'NONE',  ( -5.999999999999999112, -2.500000000000047518, 9.999999999999998224 ) ) ;
#13173=CARTESIAN_POINT ( 'NONE',  ( 0.000000000000000000, 4.999999999999999112, 0.000000000000000000 ) ) ;
#13179=ADVANCED_FACE ( 'NONE', ( #2478 ), #16910, .T. ) ;
#13181=ADVANCED_FACE ( 'NONE', ( #1134 ), #8967, .T. ) ;
#13182=CARTESIAN_POINT ( 'NONE',  ( 20.00000000000000000, 2.500000000000003997, 2.000000000000000000 ) ) ;
#13185=CARTESIAN_POINT ( 'NONE',  ( -15.61404127825609223, 0.000000000000000000, 1.000000000000000000 ) ) ;
#13187=LINE ( 'NONE', #19583, #7307 ) ;
#13194=DIRECTION ( 'NONE',  ( -0.000000000000000000, -0.000000000000000000, -1.000000000000000000 ) ) ;
#13206=ORIENTED_EDGE ( 'NONE', *, *, #11102, .T. ) ;
#13227=DIRECTION ( 'NONE',  ( -1.000000000000000000, -0.000000000000000000, 0.000000000000000000 ) ) ;
#13231=ORIENTED_EDGE ( 'NONE', *, *, #14598, .F. ) ;
#13242=EDGE_CURVE ( 'NONE', #13516, #14875, #912, .T. ) ;
#13244=CARTESIAN_POINT ( 'NONE',  ( 10.05565079891005631, 0.000000000000000000, 0.000000000000000000 ) ) ;
#13252=CARTESIAN_POINT ( 'NONE',  ( 4.247260319564023945, 9.000000000000001776, 0.000000000000000000 ) ) ;
#13254=ORIENTED_EDGE ( 'NONE', *, *, #3339, .F. ) ;
#13256=ORIENTED_EDGE ( 'NONE', *, *, #7858, .T. ) ;
#13260=LINE ( 'NONE', #2083, #7638 ) ;
#13265=DIRECTION ( 'NONE',  ( -0.000000000000000000, -0.000000000000000000, -1.000000000000000000 ) ) ;
#13273=VERTEX_POINT ( 'NONE', #11890 ) ;
#13279=CARTESIAN_POINT ( 'NONE',  ( 4.247260319564023945, 4.999999999999999112, 1.000000000000000000 ) ) ;
#13282=LINE ( 'NONE', #10259, #5631 ) ;
#13286=DIRECTION ( 'NONE',  ( -1.000000000000000000, 0.000000000000000000, 0.000000000000000000 ) ) ;
#13298=EDGE_LOOP ( 'NONE', ( #16374, #4020, #19707, #12378 ) ) ;
#13301=CARTESIAN_POINT ( 'NONE',  ( 11.49178095869207006, 9.000000000000001776, 1.000000000000000000 ) ) ;
#13310=VECTOR ( 'NONE', #10547, 1000.000000000000000 ) ;
#13311=CARTESIAN_POINT ( 'NONE',  ( -3.997260319564023501, 4.999999999999999112, 1.000000000000000000 ) ) ;
#13315=FACE_OUTER_BOUND ( 'NONE', #2406, .T. ) ;
#13316=EDGE_CURVE ( 'NONE', #4979, #14879, #3946, .T. ) ;
#13329=ORIENTED_EDGE ( 'NONE', *, *, #17901, .F. ) ;
#13331=CARTESIAN_POINT ( 'NONE',  ( 0.000000000000000000, 4.999999999999999112, 0.000000000000000000 ) ) ;
#13334=ORIENTED_EDGE ( 'NONE', *, *, #12986, .F. ) ;
#13335=DIRECTION ( 'NONE',  ( 1.000000000000000000, 0.000000000000000000, 0.000000000000000000 ) ) ;
#13337=DIRECTION ( 'NONE',  ( 0.000000000000000000, -1.000000000000000000, 0.000000000000000000 ) ) ;
#13338=EDGE_CURVE ( 'NONE', #9694, #17227, #7412, .T. ) ;
#13341=CARTESIAN_POINT ( 'NONE',  ( -21.42243175760212637, 9.000000000000001776, 1.000000000000000000 ) ) ;
#13351=EDGE_CURVE ( 'NONE', #2248, #15703, #10540, .T. ) ;
#13354=VERTEX_POINT ( 'NONE', #20176 ) ;
#13359=PLANE ( 'NONE',  #19366 ) ;
#13366=PLANE ( 'NONE',  #304 ) ;
#13371=DIRECTION ( 'NONE',  ( 0.000000000000000000, 1.000000000000000000, 0.000000000000000000 ) ) ;
#13372=DIRECTION ( 'NONE',  ( -0.000000000000000000, -0.000000000000000000, -1.000000000000000000 ) ) ;
#13380=DIRECTION ( 'NONE',  ( -0.000000000000000000, 0.000000000000000000, -1.000000000000000000 ) ) ;
#13383=CARTESIAN_POINT ( 'NONE',  ( 11.99178095869207006, 0.000000000000000000, 1.000000000000000000 ) ) ;
#13384=ORIENTED_EDGE ( 'NONE', *, *, #195, .F. ) ;
#13389=LINE ( 'NONE', #16623, #427 ) ;
#13392=CARTESIAN_POINT ( 'NONE',  ( 17.80017143803810242, 0.000000000000000000, 1.000000000000000000 ) ) ;
#13393=AXIS2_PLACEMENT_3D ( 'NONE', #9978, #11550, #3598 ) ;
#13400=LINE ( 'NONE', #14095, #15863 ) ;
#13401=LINE ( 'NONE', #10168, #8731 ) ;
#13403=EDGE_CURVE ( 'NONE', #1458, #458, #15552, .T. ) ;
#13413=ORIENTED_EDGE ( 'NONE', *, *, #2254, .T. ) ;
#13414=ORIENTED_EDGE ( 'NONE', *, *, #17526, .F. ) ;
#13424=CARTESIAN_POINT ( 'NONE',  ( -15.61404127825609223, 9.000000000000001776, 1.000000000000000000 ) ) ;
#13427=ORIENTED_EDGE ( 'NONE', *, *, #732, .T. ) ;
#13429=AXIS2_PLACEMENT_3D ( 'NONE', #16325, #8485, #19893 ) ;
#13437=ORIENTED_EDGE ( 'NONE', *, *, #10759, .T. ) ;
#13440=VERTEX_POINT ( 'NONE', #15956 ) ;
#13446=CARTESIAN_POINT ( 'NONE',  ( 2.311130159782011972, 0.000000000000000000, 1.000000000000000000 ) ) ;
#13452=DIRECTION ( 'NONE',  ( 0.000000000000000000, 1.000000000000000000, 0.000000000000000000 ) ) ;
#13464=ORIENTED_EDGE ( 'NONE', *, *, #4912, .T. ) ;
#13467=CARTESIAN_POINT ( 'NONE',  ( -13.50000000000000178, 0.000000000000000000, 1.000000000000000000 ) ) ;
#13468=ORIENTED_EDGE ( 'NONE', *, *, #20628, .T. ) ;
#13469=EDGE_CURVE ( 'NONE', #5573, #14252, #20380, .T. ) ;
#13474=LINE ( 'NONE', #8567, #3143 ) ;
#13487=LINE ( 'NONE', #2294, #18344 ) ;
#13491=VECTOR ( 'NONE', #10399, 1000.000000000000000 ) ;
#13495=DIRECTION ( 'NONE',  ( 1.000000000000000000, 0.000000000000000000, 0.000000000000000000 ) ) ;
#13502=DIRECTION ( 'NONE',  ( -0.000000000000000000, -0.000000000000000000, -1.000000000000000000 ) ) ;
#13505=DIRECTION ( 'NONE',  ( 1.000000000000000000, 0.000000000000000000, 0.000000000000000000 ) ) ;
#13516=VERTEX_POINT ( 'NONE', #19123 ) ;
#13525=DIRECTION ( 'NONE',  ( -0.000000000000000000, -0.000000000000000000, -1.000000000000000000 ) ) ;
#13539=VECTOR ( 'NONE', #17276, 1000.000000000000000 ) ;
#13546=CARTESIAN_POINT ( 'NONE',  ( -11.24178095869206828, 4.999999999999999112, 1.000000000000000000 ) ) ;
#13547=ADVANCED_FACE ( 'NONE', ( #9177 ), #20491, .F. ) ;
#13560=ORIENTED_EDGE ( 'NONE', *, *, #20280, .T. ) ;
#13565=ORIENTED_EDGE ( 'NONE', *, *, #8488, .F. ) ;
#13572=DIRECTION ( 'NONE',  ( 0.4999999999999950040, -0.8660254037844415942, 0.000000000000000000 ) ) ;
#13584=CARTESIAN_POINT ( 'NONE',  ( -17.55017143803810242, 0.000000000000000000, 1.000000000000000000 ) ) ;
#13585=ORIENTED_EDGE ( 'NONE', *, *, #1166, .F. ) ;
#13596=FACE_OUTER_BOUND ( 'NONE', #16977, .T. ) ;
#13598=CARTESIAN_POINT ( 'NONE',  ( -13.67791111847408025, 0.000000000000000000, 0.000000000000000000 ) ) ;
#13600=DIRECTION ( 'NONE',  ( 0.000000000000000000, 1.000000000000000000, 0.000000000000000000 ) ) ;
#13605=EDGE_CURVE ( 'NONE', #13273, #607, #3724, .T. ) ;
#13612=ORIENTED_EDGE ( 'NONE', *, *, #8976, .T. ) ;
#13621=LINE ( 'NONE', #15406, #17846 ) ;
#13623=CARTESIAN_POINT ( 'NONE',  ( -4.999999999999998224, 0.000000000000000000, 9.999999999999998224 ) ) ;
#13636=AXIS2_PLACEMENT_3D ( 'NONE', #7725, #8030, #16084 ) ;
#13639=ORIENTED_EDGE ( 'NONE', *, *, #417, .F. ) ;
#13643=DIRECTION ( 'NONE',  ( 0.000000000000000000, -1.000000000000000000, 0.000000000000000000 ) ) ;
#13647=LINE ( 'NONE', #15326, #9860 ) ;
#13651=CARTESIAN_POINT ( 'NONE',  ( 0.000000000000000000, 9.000000000000000000, 0.000000000000000000 ) ) ;
#13653=DIRECTION ( 'NONE',  ( 0.000000000000000000, -1.000000000000000000, 0.000000000000000000 ) ) ;
#13660=ORIENTED_EDGE ( 'NONE', *, *, #16581, .T. ) ;
#13663=ORIENTED_EDGE ( 'NONE', *, *, #4983, .F. ) ;
#13666=AXIS2_PLACEMENT_3D ( 'NONE', #15341, #12585, #8105 ) ;
#13668=ORIENTED_EDGE ( 'NONE', *, *, #11946, .F. ) ;
#13673=LINE ( 'NONE', #13784, #6639 ) ;
#13679=VERTEX_POINT ( 'NONE', #14905 ) ;
#13683=VECTOR ( 'NONE', #14629, 1000.000000000000000 ) ;
#13684=ADVANCED_FACE ( 'NONE', ( #6962 ), #19534, .T. ) ;
#13686=PLANE ( 'NONE',  #19688 ) ;
#13687=ORIENTED_EDGE ( 'NONE', *, *, #7123, .F. ) ;
#13688=VERTEX_POINT ( 'NONE', #14702 ) ;
#13691=ORIENTED_EDGE ( 'NONE', *, *, #3557, .F. ) ;
#13692=LINE ( 'NONE', #12136, #7795 ) ;
#13694=AXIS2_PLACEMENT_3D ( 'NONE', #5746, #825, #2487 ) ;
#13700=CARTESIAN_POINT ( 'NONE',  ( 0.000000000000000000, 9.000000000000001776, 1.000000000000000000 ) ) ;
#13703=VECTOR ( 'NONE', #10307, 1000.000000000000000 ) ;
#13708=DIRECTION ( 'NONE',  ( 0.000000000000000000, 0.000000000000000000, 1.000000000000000000 ) ) ;
#13710=EDGE_CURVE ( 'NONE', #20155, #3140, #1748, .T. ) ;
#13719=AXIS2_PLACEMENT_3D ( 'NONE', #340, #18122, #6724 ) ;
#13722=VECTOR ( 'NONE', #13335, 1000.000000000000000 ) ;
#13726=ADVANCED_FACE ( 'NONE', ( #8131 ), #11468, .T. ) ;
#13729=LINE ( 'NONE', #18767, #5814 ) ;
#13730=VECTOR ( 'NONE', #1991, 1000.000000000000000 ) ;
#13731=PLANE ( 'NONE',  #54 ) ;
#13732=VECTOR ( 'NONE', #18637, 1000.000000000000000 ) ;
#13736=ORIENTED_EDGE ( 'NONE', *, *, #10378, .F. ) ;
#13739=EDGE_CURVE ( 'NONE', #4438, #15088, #17850, .T. ) ;
#13742=ORIENTED_EDGE ( 'NONE', *, *, #7098, .T. ) ;
#13748=LINE ( 'NONE', #7486, #10775 ) ;
#13750=ORIENTED_EDGE ( 'NONE', *, *, #195, .T. ) ;
#13752=VECTOR ( 'NONE', #14101, 1000.000000000000000 ) ;
#13753=VERTEX_POINT ( 'NONE', #9996 ) ;
#13754=CARTESIAN_POINT ( 'NONE',  ( -24.50000000000000000, 0.000000000000000000, 0.000000000000000000 ) ) ;
#13759=DIRECTION ( 'NONE',  ( 0.000000000000000000, -1.000000000000000000, 0.000000000000000000 ) ) ;
#13762=FACE_OUTER_BOUND ( 'NONE', #18110, .T. ) ;
#13773=DIRECTION ( 'NONE',  ( -0.000000000000000000, -0.000000000000000000, -1.000000000000000000 ) ) ;
#13778=ORIENTED_EDGE ( 'NONE', *, *, #13351, .T. ) ;
#13783=DIRECTION ( 'NONE',  ( 1.000000000000000000, 0.000000000000000000, 0.000000000000000000 ) ) ;
#13784=CARTESIAN_POINT ( 'NONE',  ( 21.67243175760212637, 0.000000000000000000, 1.000000000000000000 ) ) ;
#13790=PRODUCT_DEFINITION ( 'UNKNOWN', '', #1696, #18236 ) ;
#13795=DIRECTION ( 'NONE',  ( 0.000000000000000000, 0.000000000000000000, 1.000000000000000000 ) ) ;
#13804=DIRECTION ( 'NONE',  ( 0.000000000000000000, -0.000000000000000000, 1.000000000000000000 ) ) ;
#13808=ADVANCED_FACE ( 'NONE', ( #11769 ), #4031, .T. ) ;
#13811=LINE ( 'NONE', #2518, #13732 ) ;
#13813=DIRECTION ( 'NONE',  ( -0.000000000000000000, -1.000000000000000000, -0.000000000000000000 ) ) ;
#13815=EDGE_CURVE ( 'NONE', #5367, #12057, #11970, .T. ) ;
#13818=VERTEX_POINT ( 'NONE', #7384 ) ;
#13822=ORIENTED_EDGE ( 'NONE', *, *, #7649, .T. ) ;
#13827=EDGE_CURVE ( 'NONE', #6861, #14893, #16677, .T. ) ;
#13828=FACE_OUTER_BOUND ( 'NONE', #259, .T. ) ;
#13830=PLANE ( 'NONE',  #20395 ) ;
#13836=ORIENTED_EDGE ( 'NONE', *, *, #16549, .T. ) ;
#13839=CARTESIAN_POINT ( 'NONE',  ( 0.000000000000000000, 9.000000000000001776, 1.000000000000000000 ) ) ;
#13842=EDGE_LOOP ( 'NONE', ( #3901, #5284, #1645, #11566 ) ) ;
#13844=CARTESIAN_POINT ( 'NONE',  ( 15.36404127825609400, 0.000000000000000000, 1.000000000000000000 ) ) ;
#13853=FACE_OUTER_BOUND ( 'NONE', #10094, .T. ) ;
#13856=EDGE_CURVE ( 'NONE', #1111, #17042, #3924, .T. ) ;
#13857=CARTESIAN_POINT ( 'NONE',  ( 0.000000000000000000, 0.000000000000000000, 1.000000000000000000 ) ) ;
#13860=VECTOR ( 'NONE', #4485, 1000.000000000000000 ) ;
#13863=CARTESIAN_POINT ( 'NONE',  ( -24.79469207716615031, 4.999999999999999112, 1.000000000000000000 ) ) ;
#13864=DIRECTION ( 'NONE',  ( -0.000000000000000000, 0.000000000000000000, -1.000000000000000000 ) ) ;
#13866=VECTOR ( 'NONE', #9189, 1000.000000000000000 ) ;
#13871=ORIENTED_EDGE ( 'NONE', *, *, #18576, .T. ) ;
#13874=ORIENTED_EDGE ( 'NONE', *, *, #14003, .F. ) ;
#13882=EDGE_CURVE ( 'NONE', #8244, #1149, #13748, .T. ) ;
#13891=FACE_OUTER_BOUND ( 'NONE', #11059, .T. ) ;
#13897=CARTESIAN_POINT ( 'NONE',  ( 0.000000000000000000, 4.999999999999999112, 1.000000000000000000 ) ) ;
#13901=DIRECTION ( 'NONE',  ( -0.000000000000000000, -0.000000000000000000, -1.000000000000000000 ) ) ;
#13902=VERTEX_POINT ( 'NONE', #2666 ) ;
#13904=ORIENTED_EDGE ( 'NONE', *, *, #19330, .F. ) ;
#13907=DIRECTION ( 'NONE',  ( -0.000000000000000000, 0.000000000000000000, 1.000000000000000000 ) ) ;
#13909=DIRECTION ( 'NONE',  ( 0.000000000000000000, 1.000000000000000000, -0.000000000000000000 ) ) ;
#13920=AXIS2_PLACEMENT_3D ( 'NONE', #19607, #18343, #11638 ) ;
#13924=ORIENTED_EDGE ( 'NONE', *, *, #18743, .F. ) ;
#13925=LINE ( 'NONE', #869, #15115 ) ;
#13930=CARTESIAN_POINT ( 'NONE',  ( -20.00000000000000000, -6.000000000000000000, 1.000000000000000000 ) ) ;
#13942=ORIENTED_EDGE ( 'NONE', *, *, #19738, .T. ) ;
#13947=CARTESIAN_POINT ( 'NONE',  ( -26.04469207716614676, 4.999999999999999112, 1.000000000000000000 ) ) ;
#13948=EDGE_CURVE ( 'NONE', #5550, #1363, #792, .T. ) ;
#13954=EDGE_LOOP ( 'NONE', ( #18448, #16081, #18856, #10979 ) ) ;
#13961=DIRECTION ( 'NONE',  ( 1.000000000000000000, 0.000000000000000000, 0.000000000000000000 ) ) ;
#13963=CARTESIAN_POINT ( 'NONE',  ( -2.061130159782011972, 9.000000000000001776, 0.000000000000000000 ) ) ;
#13977=ORIENTED_EDGE ( 'NONE', *, *, #9541, .T. ) ;
#13980=PLANE ( 'NONE',  #16992 ) ;
#13981=CARTESIAN_POINT ( 'NONE',  ( 17.30017143803810242, 4.999999999999999112, 0.000000000000000000 ) ) ;
#14001=AXIS2_PLACEMENT_3D ( 'NONE', #11793, #11685, #18183 ) ;
#14003=EDGE_CURVE ( 'NONE', #15372, #3140, #18884, .T. ) ;
#14009=ORIENTED_EDGE ( 'NONE', *, *, #8139, .F. ) ;
#14021=VECTOR ( 'NONE', #9929, 1000.000000000000000 ) ;
#14022=CARTESIAN_POINT ( 'NONE',  ( 0.000000000000000000, 0.000000000000000000, 1.000000000000000000 ) ) ;
#14031=ORIENTED_EDGE ( 'NONE', *, *, #4034, .F. ) ;
#14032=LINE ( 'NONE', #15598, #19476 ) ;
#14040=LINE ( 'NONE', #12476, #19394 ) ;
#14046=DIRECTION ( 'NONE',  ( 0.000000000000000000, -0.000000000000000000, 1.000000000000000000 ) ) ;
#14054=VERTEX_POINT ( 'NONE', #5031 ) ;
#14055=ORIENTED_EDGE ( 'NONE', *, *, #11197, .T. ) ;
#14062=DIRECTION ( 'NONE',  ( 0.7071067811865474617, -0.000000000000000000, -0.7071067811865474617 ) ) ;
#14063=VECTOR ( 'NONE', #11834, 1000.000000000000000 ) ;
#14065=LINE ( 'NONE', #18792, #1971 ) ;
#14072=LINE ( 'NONE', #13651, #1028 ) ;
#14080=CARTESIAN_POINT ( 'NONE',  ( -20.92243175760212637, 4.999999999999999112, 1.000000000000000000 ) ) ;
#14082=EDGE_CURVE ( 'NONE', #6097, #13688, #14547, .T. ) ;
#14084=DIRECTION ( 'NONE',  ( -0.000000000000000000, 1.000000000000000000, -0.000000000000000000 ) ) ;
#14085=EDGE_LOOP ( 'NONE', ( #13668, #6236, #4080, #15051 ) ) ;
#14091=CARTESIAN_POINT ( 'NONE',  ( -11.24178095869206828, 4.999999999999999112, 0.000000000000000000 ) ) ;
#14092=CARTESIAN_POINT ( 'NONE',  ( -9.305650798910056309, 0.000000000000000000, 1.000000000000000000 ) ) ;
#14093=VECTOR ( 'NONE', #13138, 1000.000000000000000 ) ;
#14095=CARTESIAN_POINT ( 'NONE',  ( -3.999999999999999112, -7.500000000000047073, 2.000000000000000000 ) ) ;
#14101=DIRECTION ( 'NONE',  ( -0.000000000000000000, -0.000000000000000000, -1.000000000000000000 ) ) ;
#14107=ORIENTED_EDGE ( 'NONE', *, *, #13827, .F. ) ;
#14109=SHAPE_REPRESENTATION_RELATIONSHIP ( 'NONE' , 'NONE' ,  #537, #15532 ) ;
#14110=EDGE_LOOP ( 'NONE', ( #1161, #6477, #1656, #19438 ) ) ;
#14112=VECTOR ( 'NONE', #12256, 1000.000000000000000 ) ;
#14116=CARTESIAN_POINT ( 'NONE',  ( 7.619520639128047002, 4.999999999999999112, 1.000000000000000000 ) ) ;
#14119=EDGE_CURVE ( 'NONE', #2052, #9026, #1209, .T. ) ;
#14121=DIRECTION ( 'NONE',  ( 1.000000000000000000, 0.000000000000000000, 0.000000000000000000 ) ) ;
#14130=VERTEX_POINT ( 'NONE', #2875 ) ;
#14133=VERTEX_POINT ( 'NONE', #10833 ) ;
#14150=CARTESIAN_POINT ( 'NONE',  ( 0.3749999999999968914, 4.999999999999999112, 1.000000000000000000 ) ) ;
#14153=ORIENTED_EDGE ( 'NONE', *, *, #15005, .T. ) ;
#14157=ORIENTED_EDGE ( 'NONE', *, *, #20652, .T. ) ;
#14161=CARTESIAN_POINT ( 'NONE',  ( -13.89292490618230147, -0.3192367551084450139, 0.9728728682520063620 ) ) ;
#14162=VERTEX_POINT ( 'NONE', #8276 ) ;
#14167=CARTESIAN_POINT ( 'NONE',  ( -9.805650798910056309, 9.000000000000001776, 0.000000000000000000 ) ) ;
#14168=LINE ( 'NONE', #17732, #17779 ) ;
#14179=ORIENTED_EDGE ( 'NONE', *, *, #15695, .T. ) ;
#14187=AXIS2_PLACEMENT_3D ( 'NONE', #15270, #16744, #16434 ) ;
#14189=CARTESIAN_POINT ( 'NONE',  ( -20.00000000000000000, 3.000000000000000888, 1.500000000000000000 ) ) ;
#14195=ORIENTED_EDGE ( 'NONE', *, *, #6171, .F. ) ;
#14201=CARTESIAN_POINT ( 'NONE',  ( -13.17791111847408025, 4.999999999999999112, 0.000000000000000000 ) ) ;
#14206=CARTESIAN_POINT ( 'NONE',  ( 0.000000000000000000, 9.000000000000001776, 1.000000000000000000 ) ) ;
#14211=FACE_OUTER_BOUND ( 'NONE', #4565, .T. ) ;
#14216=VECTOR ( 'NONE', #3630, 1000.000000000000000 ) ;
#14223=ORIENTED_EDGE ( 'NONE', *, *, #3216, .F. ) ;
#14225=DIRECTION ( 'NONE',  ( -1.000000000000000000, 0.000000000000000000, 0.000000000000000000 ) ) ;
#14226=ORIENTED_EDGE ( 'NONE', *, *, #17638, .F. ) ;
#14227=ADVANCED_FACE ( 'NONE', ( #3563 ), #9943, .T. ) ;
#14228=ORIENTED_EDGE ( 'NONE', *, *, #19502, .T. ) ;
#14243=DIRECTION ( 'NONE',  ( 1.000000000000000000, 0.000000000000000000, 0.000000000000000000 ) ) ;
#14249=PLANE ( 'NONE',  #4656 ) ;
#14250=ORIENTED_EDGE ( 'NONE', *, *, #14858, .T. ) ;
#14252=VERTEX_POINT ( 'NONE', #13182 ) ;
#14254=CARTESIAN_POINT ( 'NONE',  ( 14.00000000000000000, 7.867487981852999499E-15, 2.000000000000000000 ) ) ;
#14262=DIRECTION ( 'NONE',  ( 0.000000000000000000, 1.000000000000000000, -0.000000000000000000 ) ) ;
#14263=VECTOR ( 'NONE', #19043, 1000.000000000000000 ) ;
#14265=EDGE_CURVE ( 'NONE', #12176, #6649, #10361, .T. ) ;
#14267=LINE ( 'NONE', #7903, #4303 ) ;
#14277=ORIENTED_EDGE ( 'NONE', *, *, #14365, .F. ) ;
#14281=FACE_OUTER_BOUND ( 'NONE', #7327, .T. ) ;
#14284=CARTESIAN_POINT ( 'NONE',  ( 0.000000000000000000, 9.000000000000000000, 1.000000000000000000 ) ) ;
#14298=ORIENTED_EDGE ( 'NONE', *, *, #16083, .F. ) ;
#14301=ORIENTED_EDGE ( 'NONE', *, *, #16581, .F. ) ;
#14304=LINE ( 'NONE', #2926, #14940 ) ;
#14306=AXIS2_PLACEMENT_3D ( 'NONE', #16062, #1523, #17737 ) ;
#14323=CARTESIAN_POINT ( 'NONE',  ( -5.433390479346035029, 0.000000000000000000, 1.000000000000000000 ) ) ;
#14328=ORIENTED_EDGE ( 'NONE', *, *, #18899, .F. ) ;
#14329=EDGE_CURVE ( 'NONE', #1636, #2453, #2199, .T. ) ;
#14331=EDGE_CURVE ( 'NONE', #16862, #5029, #17998, .T. ) ;
#14335=DIRECTION ( 'NONE',  ( -1.734723475976807094E-15, -1.000000000000000000, 0.000000000000000000 ) ) ;
#14342=CARTESIAN_POINT ( 'NONE',  ( -27.50000000000000355, 3.000000000000000888, 0.000000000000000000 ) ) ;
#14347=DIRECTION ( 'NONE',  ( 1.000000000000000000, 0.000000000000000000, 0.000000000000000000 ) ) ;
#14351=EDGE_LOOP ( 'NONE', ( #1916, #10603, #9413, #6349 ) ) ;
#14356=MECHANICAL_DESIGN_GEOMETRIC_PRESENTATION_REPRESENTATION('',(#2005),#16704);
#14357=ORIENTED_EDGE ( 'NONE', *, *, #1560, .F. ) ;
#14360=FACE_OUTER_BOUND ( 'NONE', #13842, .T. ) ;
#14361=VERTEX_POINT ( 'NONE', #11819 ) ;
#14363=ORIENTED_EDGE ( 'NONE', *, *, #4048, .T. ) ;
#14365=EDGE_CURVE ( 'NONE', #11436, #7048, #10251, .T. ) ;
#14371=DIRECTION ( 'NONE',  ( 0.000000000000000000, -1.000000000000000000, 0.000000000000000000 ) ) ;
#14372=CARTESIAN_POINT ( 'NONE',  ( 20.00000000000000000, 0.000000000000000000, 1.000000000000000000 ) ) ;
#14373=AXIS2_PLACEMENT_3D ( 'NONE', #578, #5184, #6859 ) ;
#14374=VECTOR ( 'NONE', #12909, 1000.000000000000000 ) ;
#14375=EDGE_CURVE ( 'NONE', #10392, #10835, #12133, .T. ) ;
#14379=EDGE_CURVE ( 'NONE', #2607, #4438, #18625, .T. ) ;
#14385=VERTEX_POINT ( 'NONE', #7329 ) ;
#14387=LINE ( 'NONE', #14080, #306 ) ;
#14393=LINE ( 'NONE', #2356, #12101 ) ;
#14399=DIRECTION ( 'NONE',  ( 0.000000000000000000, 0.000000000000000000, 1.000000000000000000 ) ) ;
#14409=CYLINDRICAL_SURFACE ( 'NONE', #1727, 0.4999999999999987232 ) ;
#14415=LINE ( 'NONE', #9304, #584 ) ;
#14418=ADVANCED_FACE ( 'NONE', ( #2408 ), #12025, .T. ) ;
#14420=ORIENTED_EDGE ( 'NONE', *, *, #16083, .T. ) ;
#14428=CARTESIAN_POINT ( 'NONE',  ( -20.00000000000000000, -6.000000000000000000, 1.000000000000000000 ) ) ;
#14433=CARTESIAN_POINT ( 'NONE',  ( 0.000000000000000000, 4.999999999999999112, 1.000000000000000000 ) ) ;
#14440=ORIENTED_EDGE ( 'NONE', *, *, #7773, .F. ) ;
#14443=DIRECTION ( 'NONE',  ( -1.000000000000000000, -0.000000000000000000, -0.000000000000000000 ) ) ;
#14447=DIRECTION ( 'NONE',  ( -0.000000000000000000, -0.000000000000000000, -1.000000000000000000 ) ) ;
#14448=PLANE ( 'NONE',  #17614 ) ;
#14456=EDGE_CURVE ( 'NONE', #19021, #14162, #8799, .T. ) ;
#14457=CARTESIAN_POINT ( 'NONE',  ( 13.50000000000000178, 7.806255641895631925E-15, 2.000000000000000000 ) ) ;
#14460=VERTEX_POINT ( 'NONE', #9104 ) ;
#14466=ORIENTED_EDGE ( 'NONE', *, *, #417, .T. ) ;
#14470=ORIENTED_EDGE ( 'NONE', *, *, #14265, .F. ) ;
#14478=CARTESIAN_POINT ( 'NONE',  ( -5.999999999999999112, -2.500000000000047518, 8.999999999999998224 ) ) ;
#14480=LINE ( 'NONE', #17513, #15531 ) ;
#14481=EDGE_CURVE ( 'NONE', #1363, #15395, #4498, .T. ) ;
#14482=CARTESIAN_POINT ( 'NONE',  ( 0.000000000000000000, 4.999999999999999112, 1.000000000000000000 ) ) ;
#14485=LINE ( 'NONE', #9676, #14374 ) ;
#14498=CARTESIAN_POINT ( 'NONE',  ( 15.36404127825609400, 0.000000000000000000, 1.000000000000000000 ) ) ;
#14499=ADVANCED_FACE ( 'NONE', ( #15167 ), #20099, .T. ) ;
#14510=EDGE_CURVE ( 'NONE', #8745, #19089, #4398, .T. ) ;
#14512=ORIENTED_EDGE ( 'NONE', *, *, #7565, .F. ) ;
#14516=ORIENTED_EDGE ( 'NONE', *, *, #2732, .T. ) ;
#14518=CARTESIAN_POINT ( 'NONE',  ( 25.04469207716615031, 9.000000000000001776, 1.000000000000000000 ) ) ;
#14519=VERTEX_POINT ( 'NONE', #20301 ) ;
#14523=EDGE_CURVE ( 'NONE', #1363, #12435, #7225, .T. ) ;
#14526=VECTOR ( 'NONE', #14764, 1000.000000000000000 ) ;
#14530=FACE_OUTER_BOUND ( 'NONE', #9684, .T. ) ;
#14541=STYLED_ITEM ( 'NONE', ( #6060 ), #10862 ) ;
#14545=EDGE_LOOP ( 'NONE', ( #20044, #3214 ) ) ;
#14547=LINE ( 'NONE', #9252, #7101 ) ;
#14549=ORIENTED_EDGE ( 'NONE', *, *, #11197, .F. ) ;
#14550=DIRECTION ( 'NONE',  ( 1.000000000000000000, 0.000000000000000000, 0.000000000000000000 ) ) ;
#14558=CARTESIAN_POINT ( 'NONE',  ( -2.061130159782011972, 4.999999999999999112, 1.000000000000000000 ) ) ;
#14561=ORIENTED_EDGE ( 'NONE', *, *, #2577, .T. ) ;
#14563=LINE ( 'NONE', #14668, #11064 ) ;
#14567=EDGE_LOOP ( 'NONE', ( #1052, #6988, #8229, #10460 ) ) ;
#14570=DIRECTION ( 'NONE',  ( -0.000000000000000000, -0.000000000000000000, -1.000000000000000000 ) ) ;
#14571=ORIENTED_EDGE ( 'NONE', *, *, #12271, .T. ) ;
#14572=VERTEX_POINT ( 'NONE', #4083 ) ;
#14575=ORIENTED_EDGE ( 'NONE', *, *, #19609, .T. ) ;
#14581=PLANE ( 'NONE',  #9971 ) ;
#14584=VERTEX_POINT ( 'NONE', #18835 ) ;
#14589=VERTEX_POINT ( 'NONE', #9509 ) ;
#14595=VERTEX_POINT ( 'NONE', #15680 ) ;
#14598=EDGE_CURVE ( 'NONE', #18281, #19766, #7936, .T. ) ;
#14599=ORIENTED_EDGE ( 'NONE', *, *, #1425, .T. ) ;
#14605=LINE ( 'NONE', #12833, #19992 ) ;
#14607=FACE_OUTER_BOUND ( 'NONE', #4455, .T. ) ;
#14609=EDGE_CURVE ( 'NONE', #2020, #8434, #14415, .T. ) ;
#14610=VERTEX_POINT ( 'NONE', #17246 ) ;
#14617=DIRECTION ( 'NONE',  ( -0.000000000000000000, -0.000000000000000000, -1.000000000000000000 ) ) ;
#14623=EDGE_CURVE ( 'NONE', #19766, #11965, #1558, .T. ) ;
#14629=DIRECTION ( 'NONE',  ( 0.000000000000000000, 1.000000000000000000, -0.000000000000000000 ) ) ;
#14634=EDGE_CURVE ( 'NONE', #14460, #5550, #14304, .T. ) ;
#14650=ORIENTED_EDGE ( 'NONE', *, *, #10142, .F. ) ;
#14657=VECTOR ( 'NONE', #4987, 1000.000000000000000 ) ;
#14658=VECTOR ( 'NONE', #295, 1000.000000000000000 ) ;
#14659=DIRECTION ( 'NONE',  ( -1.000000000000000000, -1.192622389734054877E-16, 0.000000000000000000 ) ) ;
#14662=VECTOR ( 'NONE', #1541, 1000.000000000000000 ) ;
#14663=CARTESIAN_POINT ( 'NONE',  ( -4.999999999999998224, -2.500000000000047518, 9.999999999999998224 ) ) ;
#14668=CARTESIAN_POINT ( 'NONE',  ( 0.000000000000000000, 4.999999999999999112, 1.000000000000000000 ) ) ;
#14681=PLANE ( 'NONE',  #12241 ) ;
#14686=VECTOR ( 'NONE', #3571, 1000.000000000000000 ) ;
#14687=LINE ( 'NONE', #565, #11706 ) ;
#14688=DIRECTION ( 'NONE',  ( 1.000000000000000000, 0.000000000000000000, -0.000000000000000000 ) ) ;
#14700=ORIENTED_EDGE ( 'NONE', *, *, #13882, .T. ) ;
#14702=CARTESIAN_POINT ( 'NONE',  ( -21.42243175760212637, 9.000000000000001776, 0.000000000000000000 ) ) ;
#14703=ORIENTED_EDGE ( 'NONE', *, *, #12843, .F. ) ;
#14705=AXIS2_PLACEMENT_3D ( 'NONE', #7922, #1448, #3018 ) ;
#14708=VECTOR ( 'NONE', #13813, 1000.000000000000000 ) ;
#14711=DIRECTION ( 'NONE',  ( 1.000000000000000000, 0.000000000000000000, 0.000000000000000000 ) ) ;
#14715=CARTESIAN_POINT ( 'NONE',  ( 0.000000000000000000, 9.000000000000001776, 0.000000000000000000 ) ) ;
#14717=EDGE_CURVE ( 'NONE', #19171, #20470, #3233, .T. ) ;
#14719=CARTESIAN_POINT ( 'NONE',  ( 13.42791111847407848, 9.000000000000001776, 1.000000000000000000 ) ) ;
#14731=VECTOR ( 'NONE', #9850, 1000.000000000000000 ) ;
#14732=VERTEX_POINT ( 'NONE', #9604 ) ;
#14733=PRODUCT_CONTEXT ( 'NONE', #15087, 'mechanical' ) ;
#14734=ORIENTED_EDGE ( 'NONE', *, *, #8922, .F. ) ;
#14736=ORIENTED_EDGE ( 'NONE', *, *, #959, .T. ) ;
#14740=CARTESIAN_POINT ( 'NONE',  ( 0.000000000000000000, 4.999999999999999112, 1.000000000000000000 ) ) ;
#14743=LINE ( 'NONE', #3763, #13683 ) ;
#14749=LINE ( 'NONE', #3660, #16753 ) ;
#14752=ORIENTED_EDGE ( 'NONE', *, *, #17333, .F. ) ;
#14764=DIRECTION ( 'NONE',  ( 0.000000000000000000, 1.000000000000000000, -0.000000000000000000 ) ) ;
#14769=CARTESIAN_POINT ( 'NONE',  ( 19.23630159782011617, 9.000000000000001776, 1.000000000000000000 ) ) ;
#14771=AXIS2_PLACEMENT_3D ( 'NONE', #11470, #17852, #6352 ) ;
#14777=EDGE_LOOP ( 'NONE', ( #12234, #1438, #10015, #2220 ) ) ;
#14780=CARTESIAN_POINT ( 'NONE',  ( 7.619520639128047002, 4.999999999999999112, 1.000000000000000000 ) ) ;
#14783=CARTESIAN_POINT ( 'NONE',  ( 8.119520639128047890, 0.000000000000000000, 1.000000000000000000 ) ) ;
#14785=LINE ( 'NONE', #5576, #3897 ) ;
#14788=PLANE ( 'NONE',  #7322 ) ;
#14791=CARTESIAN_POINT ( 'NONE',  ( 15.86404127825609400, 0.000000000000000000, 1.000000000000000000 ) ) ;
#14792=PLANE ( 'NONE',  #13393 ) ;
#14805=LINE ( 'NONE', #6764, #4371 ) ;
#14810=CARTESIAN_POINT ( 'NONE',  ( 13.92791111847407848, 0.000000000000000000, 0.000000000000000000 ) ) ;
#14811=AXIS2_PLACEMENT_3D ( 'NONE', #17781, #107, #6493 ) ;
#14816=DIRECTION ( 'NONE',  ( 1.000000000000000000, 0.000000000000000000, 0.000000000000000000 ) ) ;
#14827=ORIENTED_EDGE ( 'NONE', *, *, #16551, .F. ) ;
#14828=EDGE_CURVE ( 'NONE', #2248, #6861, #17977, .T. ) ;
#14829=CARTESIAN_POINT ( 'NONE',  ( 1.811130159782011528, 9.000000000000001776, 1.000000000000000000 ) ) ;
#14830=LINE ( 'NONE', #7201, #9333 ) ;
#14839=CARTESIAN_POINT ( 'NONE',  ( 13.50000000000000178, 7.806255641895631925E-15, 1.000000000000000000 ) ) ;
#14841=DIRECTION ( 'NONE',  ( 0.000000000000000000, -0.000000000000000000, -1.000000000000000000 ) ) ;
#14846=CARTESIAN_POINT ( 'NONE',  ( 13.42791111847407848, 4.999999999999999112, 1.000000000000000000 ) ) ;
#14847=EDGE_CURVE ( 'NONE', #15883, #8680, #13260, .T. ) ;
#14858=EDGE_CURVE ( 'NONE', #1213, #9491, #3853, .T. ) ;
#14864=CARTESIAN_POINT ( 'NONE',  ( 25.04469207716615031, 0.000000000000000000, 0.000000000000000000 ) ) ;
#14875=VERTEX_POINT ( 'NONE', #10232 ) ;
#14879=VERTEX_POINT ( 'NONE', #3755 ) ;
#14881=CYLINDRICAL_SURFACE ( 'NONE', #7450, 2.999999999999999112 ) ;
#14884=ADVANCED_FACE ( 'NONE', ( #11897 ), #13366, .F. ) ;
#14888=CARTESIAN_POINT ( 'NONE',  ( -5.999999999999999112, -2.500000000000047518, 2.000000000000000000 ) ) ;
#14893=VERTEX_POINT ( 'NONE', #6999 ) ;
#14899=ORIENTED_EDGE ( 'NONE', *, *, #5885, .F. ) ;
#14902=DIRECTION ( 'NONE',  ( -0.000000000000000000, -0.000000000000000000, -1.000000000000000000 ) ) ;
#14905=CARTESIAN_POINT ( 'NONE',  ( -3.497260319564023057, 4.999999999999999112, 0.000000000000000000 ) ) ;
#14912=DIRECTION ( 'NONE',  ( -1.000000000000000000, 0.000000000000000000, 0.000000000000000000 ) ) ;
#14928=ORIENTED_EDGE ( 'NONE', *, *, #8519, .F. ) ;
#14933=LINE ( 'NONE', #16306, #924 ) ;
#14940=VECTOR ( 'NONE', #11183, 1000.000000000000000 ) ;
#14949=ORIENTED_EDGE ( 'NONE', *, *, #9673, .F. ) ;
#14953=ORIENTED_EDGE ( 'NONE', *, *, #16436, .T. ) ;
#14954=DIRECTION ( 'NONE',  ( 1.000000000000000000, 0.000000000000000000, 0.000000000000000000 ) ) ;
#14955=CARTESIAN_POINT ( 'NONE',  ( 5.999999999999999112, -7.500000000000047073, 8.999999999999998224 ) ) ;
#14957=FACE_OUTER_BOUND ( 'NONE', #6346, .T. ) ;
#14959=PLANE ( 'NONE',  #15542 ) ;
#14965=CARTESIAN_POINT ( 'NONE',  ( 1.811130159782011528, 0.000000000000000000, 0.000000000000000000 ) ) ;
#14971=EDGE_CURVE ( 'NONE', #6994, #18278, #9181, .T. ) ;
#14976=AXIS2_PLACEMENT_3D ( 'NONE', #18912, #4570, #15757 ) ;
#14986=ADVANCED_FACE ( 'NONE', ( #7305 ), #13980, .T. ) ;
#14990=LINE ( 'NONE', #8518, #18081 ) ;
#14992=CARTESIAN_POINT ( 'NONE',  ( 0.000000000000000000, 4.999999999999999112, 1.000000000000000000 ) ) ;
#14995=VECTOR ( 'NONE', #15095, 1000.000000000000000 ) ;
#15005=EDGE_CURVE ( 'NONE', #999, #4851, #10648, .T. ) ;
#15008=VERTEX_POINT ( 'NONE', #7418 ) ;
#15010=ORIENTED_EDGE ( 'NONE', *, *, #5398, .T. ) ;
#15014=VECTOR ( 'NONE', #17823, 1000.000000000000000 ) ;
#15015=EDGE_CURVE ( 'NONE', #11469, #19731, #7517, .T. ) ;
#15031=CYLINDRICAL_SURFACE ( 'NONE', #14001, 0.5000000000000000000 ) ;
#15034=VERTEX_POINT ( 'NONE', #10757 ) ;
#15035=AXIS2_PLACEMENT_3D ( 'NONE', #60, #14688, #369 ) ;
#15036=CARTESIAN_POINT ( 'NONE',  ( -14.00000000000000355, -9.599706735548742312E-18, 0.5896324317178637253 ) ) ;
#15042=CARTESIAN_POINT ( 'NONE',  ( -3.497260319564023057, 4.999999999999999112, 1.000000000000000000 ) ) ;
#15044=CARTESIAN_POINT ( 'NONE',  ( -17.11324865405191176, -11.00000000000000000, 1.000000000000000000 ) ) ;
#15051=ORIENTED_EDGE ( 'NONE', *, *, #4304, .T. ) ;
#15055=ADVANCED_FACE ( 'NONE', ( #7613 ), #15454, .T. ) ;
#15063=LINE ( 'NONE', #16430, #4450 ) ;
#15065=CARTESIAN_POINT ( 'NONE',  ( 0.000000000000000000, 4.999999999999999112, 0.000000000000000000 ) ) ;
#15078=AXIS2_PLACEMENT_3D ( 'NONE', #11904, #13371, #12402 ) ;
#15084=CARTESIAN_POINT ( 'NONE',  ( -11.24178095869206828, 0.000000000000000000, 1.000000000000000000 ) ) ;
#15087=APPLICATION_CONTEXT ( 'automotive_design' ) ;
#15088=VERTEX_POINT ( 'NONE', #5742 ) ;
#15094=VECTOR ( 'NONE', #7993, 1000.000000000000000 ) ;
#15095=DIRECTION ( 'NONE',  ( 0.000000000000000000, -1.000000000000000000, 0.000000000000000000 ) ) ;
#15097=CARTESIAN_POINT ( 'NONE',  ( 0.000000000000000000, 0.000000000000000000, 1.000000000000000000 ) ) ;
#15099=VECTOR ( 'NONE', #12674, 1000.000000000000000 ) ;
#15115=VECTOR ( 'NONE', #20326, 1000.000000000000000 ) ;
#15121=ADVANCED_FACE ( 'NONE', ( #17127 ), #2907, .F. ) ;
#15122=ORIENTED_EDGE ( 'NONE', *, *, #18999, .F. ) ;
#15123=CARTESIAN_POINT ( 'NONE',  ( -5.433390479346035029, 9.000000000000001776, 1.000000000000000000 ) ) ;
#15124=CARTESIAN_POINT ( 'NONE',  ( 5.999999999999999112, -2.500000000000047518, 8.999999999999998224 ) ) ;
#15133=CARTESIAN_POINT ( 'NONE',  ( -24.79469207716615031, 0.000000000000000000, 0.000000000000000000 ) ) ;
#15139=ORIENTED_EDGE ( 'NONE', *, *, #3761, .T. ) ;
#15146=ORIENTED_EDGE ( 'NONE', *, *, #3524, .F. ) ;
#15148=FACE_OUTER_BOUND ( 'NONE', #18184, .T. ) ;
#15152=EDGE_CURVE ( 'NONE', #12662, #3823, #15860, .T. ) ;
#15157=EDGE_LOOP ( 'NONE', ( #8022, #11968, #13612, #5741 ) ) ;
#15162=EDGE_CURVE ( 'NONE', #5259, #8157, #8136, .T. ) ;
#15163=FACE_OUTER_BOUND ( 'NONE', #14567, .T. ) ;
#15165=EDGE_LOOP ( 'NONE', ( #11162, #11916, #20587, #16144 ) ) ;
#15167=FACE_OUTER_BOUND ( 'NONE', #7265, .T. ) ;
#15171=LINE ( 'NONE', #10056, #9028 ) ;
#15172=LINE ( 'NONE', #18215, #1309 ) ;
#15174=CARTESIAN_POINT ( 'NONE',  ( 23.60856191738414012, 4.999999999999999112, 0.000000000000000000 ) ) ;
#15189=LINE ( 'NONE', #15497, #335 ) ;
#15192=CARTESIAN_POINT ( 'NONE',  ( 25.54469207716615031, 4.999999999999999112, 1.000000000000000000 ) ) ;
#15200=LINE ( 'NONE', #8929, #1714 ) ;
#15213=ORIENTED_EDGE ( 'NONE', *, *, #12162, .F. ) ;
#15215=ORIENTED_EDGE ( 'NONE', *, *, #4716, .F. ) ;
#15220=CARTESIAN_POINT ( 'NONE',  ( 17.80017143803810242, 4.999999999999999112, 0.000000000000000000 ) ) ;
#15226=EDGE_CURVE ( 'NONE', #9491, #13688, #9900, .T. ) ;
#15228=DIRECTION ( 'NONE',  ( -0.000000000000000000, -0.000000000000000000, -1.000000000000000000 ) ) ;
#15234=VERTEX_POINT ( 'NONE', #5192 ) ;
#15239=ADVANCED_FACE ( 'NONE', ( #799 ), #11773, .T. ) ;
#15244=ORIENTED_EDGE ( 'NONE', *, *, #16361, .T. ) ;
#15248=DIRECTION ( 'NONE',  ( -0.000000000000000000, -0.000000000000000000, -1.000000000000000000 ) ) ;
#15255=VERTEX_POINT ( 'NONE', #15123 ) ;
#15257=CARTESIAN_POINT ( 'NONE',  ( -17.55017143803810242, 9.000000000000001776, 0.000000000000000000 ) ) ;
#15264=DIRECTION ( 'NONE',  ( 0.000000000000000000, -1.000000000000000000, 0.000000000000000000 ) ) ;
#15265=EDGE_LOOP ( 'NONE', ( #8201, #15628, #3128, #18756 ) ) ;
#15268=DIRECTION ( 'NONE',  ( -0.000000000000000000, 0.000000000000000000, -1.000000000000000000 ) ) ;
#15270=CARTESIAN_POINT ( 'NONE',  ( 0.000000000000000000, 9.000000000000001776, 1.000000000000000000 ) ) ;
#15274=ADVANCED_FACE ( 'NONE', ( #4038 ), #7281, .T. ) ;
#15280=PLANE ( 'NONE',  #7718 ) ;
#15286=LINE ( 'NONE', #15084, #17019 ) ;
#15290=ORIENTED_EDGE ( 'NONE', *, *, #5819, .T. ) ;
#15299=PLANE ( 'NONE',  #15739 ) ;
#15300=VECTOR ( 'NONE', #14084, 1000.000000000000000 ) ;
#15311=CARTESIAN_POINT ( 'NONE',  ( 0.000000000000000000, 9.000000000000001776, 1.000000000000000000 ) ) ;
#15312=ORIENTED_EDGE ( 'NONE', *, *, #6279, .T. ) ;
#15314=EDGE_CURVE ( 'NONE', #16322, #13679, #4139, .T. ) ;
#15320=CARTESIAN_POINT ( 'NONE',  ( -3.497260319564023057, 4.999999999999999112, 1.000000000000000000 ) ) ;
#15321=LINE ( 'NONE', #19948, #19702 ) ;
#15326=CARTESIAN_POINT ( 'NONE',  ( -7.369520639128046113, 0.000000000000000000, 1.000000000000000000 ) ) ;
#15330=DIRECTION ( 'NONE',  ( -0.000000000000000000, -0.000000000000000000, -1.000000000000000000 ) ) ;
#15336=VERTEX_POINT ( 'NONE', #895 ) ;
#15339=ORIENTED_EDGE ( 'NONE', *, *, #17030, .F. ) ;
#15340=DIRECTION ( 'NONE',  ( 0.000000000000000000, 0.000000000000000000, 1.000000000000000000 ) ) ;
#15341=CARTESIAN_POINT ( 'NONE',  ( 0.000000000000000000, 4.999999999999999112, 1.000000000000000000 ) ) ;
#15345=ORIENTED_EDGE ( 'NONE', *, *, #3340, .T. ) ;
#15346=EDGE_CURVE ( 'NONE', #14595, #15669, #20359, .T. ) ;
#15354=CARTESIAN_POINT ( 'NONE',  ( 7.619520639128047002, 9.000000000000001776, 0.000000000000000000 ) ) ;
#15367=CARTESIAN_POINT ( 'NONE',  ( 0.000000000000000000, 0.000000000000000000, 1.000000000000000000 ) ) ;
#15369=ORIENTED_EDGE ( 'NONE', *, *, #15577, .F. ) ;
#15372=VERTEX_POINT ( 'NONE', #1115 ) ;
#15373=ADVANCED_FACE ( 'NONE', ( #13853 ), #2462, .T. ) ;
#15375=VECTOR ( 'NONE', #17182, 1000.000000000000000 ) ;
#15377=ORIENTED_EDGE ( 'NONE', *, *, #3593, .T. ) ;
#15382=AXIS2_PLACEMENT_3D ( 'NONE', #8127, #13227, #19531 ) ;
#15383=VECTOR ( 'NONE', #5923, 1000.000000000000000 ) ;
#15395=VERTEX_POINT ( 'NONE', #15220 ) ;
#15398=ORIENTED_EDGE ( 'NONE', *, *, #16071, .T. ) ;
#15400=CARTESIAN_POINT ( 'NONE',  ( 26.04469207716615031, 0.000000000000000000, 1.000000000000000000 ) ) ;
#15406=CARTESIAN_POINT ( 'NONE',  ( 2.311130159782011972, 4.999999999999999112, 1.000000000000000000 ) ) ;
#15409=VECTOR ( 'NONE', #1707, 1000.000000000000000 ) ;
#15415=PLANE ( 'NONE',  #18410 ) ;
#15420=FACE_OUTER_BOUND ( 'NONE', #18422, .T. ) ;
#15422=VERTEX_POINT ( 'NONE', #13754 ) ;
#15425=EDGE_LOOP ( 'NONE', ( #17049, #3565, #5004, #9800 ) ) ;
#15426=EDGE_CURVE ( 'NONE', #1844, #4979, #17204, .T. ) ;
#15429=CARTESIAN_POINT ( 'NONE',  ( -3.497260319564023057, 0.000000000000000000, 0.000000000000000000 ) ) ;
#15434=PLANE ( 'NONE',  #983 ) ;
#15439=LINE ( 'NONE', #1426, #20351 ) ;
#15440=LINE ( 'NONE', #9167, #19744 ) ;
#15446=ORIENTED_EDGE ( 'NONE', *, *, #3222, .T. ) ;
#15449=ORIENTED_EDGE ( 'NONE', *, *, #4954, .T. ) ;
#15454=PLANE ( 'NONE',  #17666 ) ;
#15455=VECTOR ( 'NONE', #9635, 1000.000000000000000 ) ;
#15460=CARTESIAN_POINT ( 'NONE',  ( -1.561130159782011306, 4.999999999999999112, 1.000000000000000000 ) ) ;
#15464=EDGE_CURVE ( 'NONE', #10048, #6813, #20156, .T. ) ;
#15465=AXIS2_PLACEMENT_3D ( 'NONE', #14740, #416, #6797 ) ;
#15466=EDGE_LOOP ( 'NONE', ( #13736, #10220, #19653, #13256 ) ) ;
#15467=CARTESIAN_POINT ( 'NONE',  ( 3.747260319564023501, 4.999999999999999112, 1.000000000000000000 ) ) ;
#15468=CARTESIAN_POINT ( 'NONE',  ( -3.997260319564023501, 4.999999999999999112, 1.000000000000000000 ) ) ;
#15470=VECTOR ( 'NONE', #4700, 1000.000000000000000 ) ;
#15473=ORIENTED_EDGE ( 'NONE', *, *, #17592, .F. ) ;
#15478=CARTESIAN_POINT ( 'NONE',  ( 23.10856191738414012, 9.000000000000001776, 0.000000000000000000 ) ) ;
#15479=ORIENTED_EDGE ( 'NONE', *, *, #13085, .F. ) ;
#15484=CARTESIAN_POINT ( 'NONE',  ( 23.10856191738414012, 4.999999999999999112, 1.000000000000000000 ) ) ;
#15489=CARTESIAN_POINT ( 'NONE',  ( -2.061130159782011972, 0.000000000000000000, 1.000000000000000000 ) ) ;
#15496=ADVANCED_FACE ( 'NONE', ( #5044 ), #6325, .T. ) ;
#15497=CARTESIAN_POINT ( 'NONE',  ( -20.00000000000000000, 0.000000000000000000, 2.000000000000000000 ) ) ;
#15500=VERTEX_POINT ( 'NONE', #15737 ) ;
#15503=CARTESIAN_POINT ( 'NONE',  ( 10.05565079891005631, 4.999999999999999112, 1.000000000000000000 ) ) ;
#15527=CARTESIAN_POINT ( 'NONE',  ( -13.58954612507874238, -0.5000000000000004441, 1.000000000000000000 ) ) ;
#15530=CARTESIAN_POINT ( 'NONE',  ( 9.555650798910054533, 4.999999999999999112, 0.000000000000000000 ) ) ;
#15531=VECTOR ( 'NONE', #159, 1000.000000000000000 ) ;
#15532=ADVANCED_BREP_SHAPE_REPRESENTATION ( '', ( #10862, #18039 ), #19052 ) ;
#15536=DIRECTION ( 'NONE',  ( 1.000000000000000000, 0.000000000000000000, 0.000000000000000000 ) ) ;
#15537=EDGE_CURVE ( 'NONE', #3029, #1688, #8394, .T. ) ;
#15538=CARTESIAN_POINT ( 'NONE',  ( 13.92791111847407848, 9.000000000000001776, 1.000000000000000000 ) ) ;
#15541=LINE ( 'NONE', #10629, #6373 ) ;
#15542=AXIS2_PLACEMENT_3D ( 'NONE', #5556, #13286, #750 ) ;
#15550=CARTESIAN_POINT ( 'NONE',  ( 15.86404127825609400, 9.000000000000001776, 1.000000000000000000 ) ) ;
#15552=LINE ( 'NONE', #19223, #17649 ) ;
#15557=CARTESIAN_POINT ( 'NONE',  ( 0.000000000000000000, 0.000000000000000000, 0.000000000000000000 ) ) ;
#15561=DIRECTION ( 'NONE',  ( 0.000000000000000000, -1.000000000000000000, 0.000000000000000000 ) ) ;
#15571=PLANE ( 'NONE',  #5316 ) ;
#15577=EDGE_CURVE ( 'NONE', #17227, #19021, #6820, .T. ) ;
#15578=DIRECTION ( 'NONE',  ( 0.000000000000000000, 1.000000000000000000, -0.000000000000000000 ) ) ;
#15579=ORIENTED_EDGE ( 'NONE', *, *, #8886, .T. ) ;
#15580=CARTESIAN_POINT ( 'NONE',  ( -0.1250000000000035805, 4.999999999999999112, 1.000000000000000000 ) ) ;
#15581=CARTESIAN_POINT ( 'NONE',  ( 15.86404127825609400, 4.999999999999999112, 0.000000000000000000 ) ) ;
#15582=DIRECTION ( 'NONE',  ( 0.000000000000000000, -1.000000000000000000, 0.000000000000000000 ) ) ;
#15584=CARTESIAN_POINT ( 'NONE',  ( -9.305650798910056309, 4.999999999999999112, 1.000000000000000000 ) ) ;
#15588=DIRECTION ( 'NONE',  ( 1.000000000000000000, 0.000000000000000000, 0.000000000000000000 ) ) ;
#15597=ORIENTED_EDGE ( 'NONE', *, *, #14082, .T. ) ;
#15598=CARTESIAN_POINT ( 'NONE',  ( 25.54469207716615031, 0.000000000000000000, 0.000000000000000000 ) ) ;
#15603=EDGE_CURVE ( 'NONE', #11770, #15422, #6222, .T. ) ;
#15604=DIRECTION ( 'NONE',  ( 0.000000000000000000, 1.000000000000000000, 0.000000000000000000 ) ) ;
#15605=CARTESIAN_POINT ( 'NONE',  ( 6.183390479346035917, 9.000000000000001776, 1.000000000000000000 ) ) ;
#15609=LINE ( 'NONE', #13623, #15645 ) ;
#15612=ORIENTED_EDGE ( 'NONE', *, *, #3626, .T. ) ;
#15617=ORIENTED_EDGE ( 'NONE', *, *, #16394, .F. ) ;
#15627=AXIS2_PLACEMENT_3D ( 'NONE', #10009, #13452, #18171 ) ;
#15628=ORIENTED_EDGE ( 'NONE', *, *, #5555, .F. ) ;
#15630=VECTOR ( 'NONE', #18595, 1000.000000000000000 ) ;
#15632=DIRECTION ( 'NONE',  ( 1.000000000000000000, 0.000000000000000000, 0.000000000000000000 ) ) ;
#15636=DIRECTION ( 'NONE',  ( 1.000000000000000000, 0.000000000000000000, 0.000000000000000000 ) ) ;
#15637=CARTESIAN_POINT ( 'NONE',  ( 4.247260319564023945, 4.999999999999999112, 0.000000000000000000 ) ) ;
#15638=DIRECTION ( 'NONE',  ( 1.000000000000000000, 0.000000000000000000, 0.000000000000000000 ) ) ;
#15645=VECTOR ( 'NONE', #20031, 1000.000000000000000 ) ;
#15658=ORIENTED_EDGE ( 'NONE', *, *, #5438, .T. ) ;
#15663=FACE_OUTER_BOUND ( 'NONE', #11945, .T. ) ;
#15664=LINE ( 'NONE', #4379, #6023 ) ;
#15667=ADVANCED_FACE ( 'NONE', ( #13596 ), #19899, .T. ) ;
#15669=VERTEX_POINT ( 'NONE', #15174 ) ;
#15677=AXIS2_PLACEMENT_3D ( 'NONE', #8871, #4059, #3749 ) ;
#15680=CARTESIAN_POINT ( 'NONE',  ( 23.60856191738414012, 4.999999999999999112, 1.000000000000000000 ) ) ;
#15681=( NAMED_UNIT ( * ) PLANE_ANGLE_UNIT ( ) SI_UNIT ( $, .RADIAN. ) );
#15687=DIRECTION ( 'NONE',  ( 0.000000000000000000, -0.000000000000000000, 1.000000000000000000 ) ) ;
#15688=DIRECTION ( 'NONE',  ( 1.000000000000000000, 0.000000000000000000, 0.000000000000000000 ) ) ;
#15695=EDGE_CURVE ( 'NONE', #10100, #9451, #2306, .T. ) ;
#15696=VECTOR ( 'NONE', #6275, 1000.000000000000000 ) ;
#15700=ORIENTED_EDGE ( 'NONE', *, *, #10950, .T. ) ;
#15703=VERTEX_POINT ( 'NONE', #2513 ) ;
#15713=CARTESIAN_POINT ( 'NONE',  ( 0.000000000000000000, 9.000000000000001776, 1.000000000000000000 ) ) ;
#15720=AXIS2_PLACEMENT_3D ( 'NONE', #15489, #2423, #13708 ) ;
#15722=LINE ( 'NONE', #16877, #695 ) ;
#15723=VECTOR ( 'NONE', #13525, 1000.000000000000000 ) ;
#15724=EDGE_CURVE ( 'NONE', #16371, #3612, #11827, .T. ) ;
#15731=PLANE ( 'NONE',  #11013 ) ;
#15736=EDGE_LOOP ( 'NONE', ( #6217, #11759, #16423, #5468 ) ) ;
#15737=CARTESIAN_POINT ( 'NONE',  ( -15.61404127825609223, 4.999999999999999112, 1.000000000000000000 ) ) ;
#15739=AXIS2_PLACEMENT_3D ( 'NONE', #7261, #17082, #4219 ) ;
#15740=CARTESIAN_POINT ( 'NONE',  ( -13.50000000000000178, 0.000000000000000000, 2.000000000000000000 ) ) ;
#15745=DIRECTION ( 'NONE',  ( 1.192622389734054384E-16, -1.000000000000000000, 0.000000000000000000 ) ) ;
#15755=ORIENTED_EDGE ( 'NONE', *, *, #16617, .T. ) ;
#15756=VECTOR ( 'NONE', #19143, 1000.000000000000000 ) ;
#15757=DIRECTION ( 'NONE',  ( 0.000000000000000000, -0.000000000000000000, 1.000000000000000000 ) ) ;
#15762=ORIENTED_EDGE ( 'NONE', *, *, #14634, .F. ) ;
#15764=PLANE ( 'NONE',  #3968 ) ;
#15766=FACE_OUTER_BOUND ( 'NONE', #1333, .T. ) ;
#15767=CARTESIAN_POINT ( 'NONE',  ( -20.92243175760212637, 0.000000000000000000, 1.000000000000000000 ) ) ;
#15768=VECTOR ( 'NONE', #5074, 1000.000000000000000 ) ;
#15769=CARTESIAN_POINT ( 'NONE',  ( 13.50000000000000178, 7.806255641895631925E-15, 1.000000000000000000 ) ) ;
#15773=ADVANCED_FACE ( 'NONE', ( #7136 ), #14959, .T. ) ;
#15774=ORIENTED_EDGE ( 'NONE', *, *, #2217, .F. ) ;
#15776=DIRECTION ( 'NONE',  ( 0.000000000000000000, 1.000000000000000000, 0.000000000000000000 ) ) ;
#15784=FILL_AREA_STYLE_COLOUR ( '', #6355 ) ;
#15785=EDGE_LOOP ( 'NONE', ( #1746, #7715, #3852, #7351 ) ) ;
#15797=AXIS2_PLACEMENT_3D ( 'NONE', #3980, #10363, #7332 ) ;
#15799=EDGE_CURVE ( 'NONE', #18810, #8332, #5349, .T. ) ;
#15804=ORIENTED_EDGE ( 'NONE', *, *, #12299, .T. ) ;
#15805=ADVANCED_FACE ( 'NONE', ( #10477 ), #16532, .T. ) ;
#15808=ORIENTED_EDGE ( 'NONE', *, *, #6279, .F. ) ;
#15809=ORIENTED_EDGE ( 'NONE', *, *, #10567, .F. ) ;
#15810=CARTESIAN_POINT ( 'NONE',  ( -27.49999999999999645, -4.770489558936219510E-14, 1.000000000000000000 ) ) ;
#15811=EDGE_CURVE ( 'NONE', #20271, #16070, #2110, .T. ) ;
#15818=LINE ( 'NONE', #10915, #15409 ) ;
#15831=CARTESIAN_POINT ( 'NONE',  ( 17.11324865405191176, -10.99999999999999645, 2.000000000000000000 ) ) ;
#15832=EDGE_LOOP ( 'NONE', ( #177, #20435, #9226, #633 ) ) ;
#15838=DIRECTION ( 'NONE',  ( 1.000000000000000000, 0.000000000000000000, 0.000000000000000000 ) ) ;
#15840=LINE ( 'NONE', #19104, #16664 ) ;
#15842=CARTESIAN_POINT ( 'NONE',  ( -24.79469207716615031, 9.000000000000001776, 0.000000000000000000 ) ) ;
#15844=DIRECTION ( 'NONE',  ( 1.000000000000000000, -0.000000000000000000, -0.000000000000000000 ) ) ;
#15860=LINE ( 'NONE', #17537, #14662 ) ;
#15863=VECTOR ( 'NONE', #13600, 1000.000000000000000 ) ;
#15868=ADVANCED_FACE ( 'NONE', ( #11727 ), #19686, .T. ) ;
#15869=EDGE_CURVE ( 'NONE', #16909, #381, #17159, .T. ) ;
#15874=ORIENTED_EDGE ( 'NONE', *, *, #8029, .F. ) ;
#15880=ORIENTED_EDGE ( 'NONE', *, *, #19670, .F. ) ;
#15881=DIRECTION ( 'NONE',  ( 0.000000000000000000, 1.000000000000000000, -0.000000000000000000 ) ) ;
#15883=VERTEX_POINT ( 'NONE', #17054 ) ;
#15884=DIRECTION ( 'NONE',  ( -0.000000000000000000, -0.000000000000000000, -1.000000000000000000 ) ) ;
#15885=EDGE_LOOP ( 'NONE', ( #20413, #10558, #3608, #12748 ) ) ;
#15888=ADVANCED_FACE ( 'NONE', ( #3044 ), #2733, .T. ) ;
#15895=DIRECTION ( 'NONE',  ( 1.000000000000000000, 0.000000000000000000, 0.000000000000000000 ) ) ;
#15897=DIRECTION ( 'NONE',  ( 0.000000000000000000, -0.000000000000000000, 1.000000000000000000 ) ) ;
#15898=EDGE_CURVE ( 'NONE', #2944, #14584, #9008, .T. ) ;
#15901=ORIENTED_EDGE ( 'NONE', *, *, #11829, .T. ) ;
#15903=DIRECTION ( 'NONE',  ( 0.000000000000000000, 0.000000000000000000, 1.000000000000000000 ) ) ;
#15904=ORIENTED_EDGE ( 'NONE', *, *, #10655, .F. ) ;
#15906=ORIENTED_EDGE ( 'NONE', *, *, #2779, .T. ) ;
#15911=EDGE_CURVE ( 'NONE', #15088, #6051, #17252, .T. ) ;
#15914=DIRECTION ( 'NONE',  ( 1.000000000000000000, 0.000000000000000000, 0.000000000000000000 ) ) ;
#15917=DIRECTION ( 'NONE',  ( 0.000000000000000000, 0.000000000000000000, 1.000000000000000000 ) ) ;
#15924=ADVANCED_FACE ( 'NONE', ( #1469 ), #10989, .T. ) ;
#15931=EDGE_LOOP ( 'NONE', ( #1794, #4719, #11682, #11786 ) ) ;
#15938=LINE ( 'NONE', #16163, #4984 ) ;
#15940=DIRECTION ( 'NONE',  ( 1.000000000000000000, 0.000000000000000000, 0.000000000000000000 ) ) ;
#15942=LINE ( 'NONE', #11242, #9016 ) ;
#15956=CARTESIAN_POINT ( 'NONE',  ( 21.67243175760212637, 9.000000000000001776, 0.000000000000000000 ) ) ;
#15957=ORIENTED_EDGE ( 'NONE', *, *, #17569, .F. ) ;
#15959=AXIS2_PLACEMENT_3D ( 'NONE', #18082, #2076, #3844 ) ;
#15962=VERTEX_POINT ( 'NONE', #4506 ) ;
#15974=VERTEX_POINT ( 'NONE', #2933 ) ;
#15976=FACE_OUTER_BOUND ( 'NONE', #18526, .T. ) ;
#15978=ORIENTED_EDGE ( 'NONE', *, *, #16904, .F. ) ;
#15981=CARTESIAN_POINT ( 'NONE',  ( 6.183390479346035917, 4.999999999999999112, 1.000000000000000000 ) ) ;
#15982=VERTEX_POINT ( 'NONE', #1065 ) ;
#15983=AXIS2_PLACEMENT_3D ( 'NONE', #16795, #801, #11669 ) ;
#15988=DIRECTION ( 'NONE',  ( 1.000000000000000000, 0.000000000000000000, 0.000000000000000000 ) ) ;
#15989=ADVANCED_FACE ( 'NONE', ( #14211 ), #12545, .T. ) ;
#15990=EDGE_CURVE ( 'NONE', #14162, #9049, #1371, .T. ) ;
#15992=ORIENTED_EDGE ( 'NONE', *, *, #14365, .T. ) ;
#15995=DIRECTION ( 'NONE',  ( 0.000000000000000000, 1.000000000000000000, 0.000000000000000000 ) ) ;
#15997=PLANE ( 'NONE',  #12725 ) ;
#16000=VECTOR ( 'NONE', #1446, 1000.000000000000000 ) ;
#16022=FACE_BOUND ( 'NONE', #16155, .T. ) ;
#16024=VECTOR ( 'NONE', #6214, 1000.000000000000000 ) ;
#16027=VECTOR ( 'NONE', #11905, 1000.000000000000000 ) ;
#16028=DIRECTION ( 'NONE',  ( 1.000000000000000000, 0.000000000000000000, 0.000000000000000000 ) ) ;
#16030=CARTESIAN_POINT ( 'NONE',  ( -24.79469207716615031, 4.999999999999999112, 1.000000000000000000 ) ) ;
#16034=ORIENTED_EDGE ( 'NONE', *, *, #13948, .T. ) ;
#16038=EDGE_CURVE ( 'NONE', #10986, #2075, #18632, .T. ) ;
#16041=VECTOR ( 'NONE', #10653, 1000.000000000000000 ) ;
#16051=LINE ( 'NONE', #13114, #16914 ) ;
#16059=CIRCLE ( 'NONE', #15382, 0.5000000000000000000 ) ;
#16061=DIRECTION ( 'NONE',  ( -0.000000000000000000, -0.000000000000000000, -1.000000000000000000 ) ) ;
#16062=CARTESIAN_POINT ( 'NONE',  ( -20.00000000000000000, 3.499999999999999556, 1.500000000000000000 ) ) ;
#16070=VERTEX_POINT ( 'NONE', #9926 ) ;
#16071=EDGE_CURVE ( 'NONE', #17458, #11469, #17467, .T. ) ;
#16079=VECTOR ( 'NONE', #4839, 1000.000000000000000 ) ;
#16081=ORIENTED_EDGE ( 'NONE', *, *, #14481, .F. ) ;
#16083=EDGE_CURVE ( 'NONE', #49, #18833, #10519, .T. ) ;
#16084=DIRECTION ( 'NONE',  ( -0.000000000000000000, 0.000000000000000000, -1.000000000000000000 ) ) ;
#16092=AXIS2_PLACEMENT_3D ( 'NONE', #3154, #9525, #15897 ) ;
#16099=DIRECTION ( 'NONE',  ( 1.000000000000000000, 1.013672804646636068E-16, 0.000000000000000000 ) ) ;
#16108=DIRECTION ( 'NONE',  ( 0.000000000000000000, -0.000000000000000000, 1.000000000000000000 ) ) ;
#16115=VECTOR ( 'NONE', #19483, 1000.000000000000000 ) ;
#16127=ORIENTED_EDGE ( 'NONE', *, *, #11154, .F. ) ;
#16129=CARTESIAN_POINT ( 'NONE',  ( 20.00000000000000000, 3.000000000000004441, 1.500000000000000000 ) ) ;
#16136=EDGE_CURVE ( 'NONE', #9411, #1583, #12955, .T. ) ;
#16137=CARTESIAN_POINT ( 'NONE',  ( 0.000000000000000000, 4.999999999999999112, 0.000000000000000000 ) ) ;
#16144=ORIENTED_EDGE ( 'NONE', *, *, #3557, .T. ) ;
#16155=EDGE_LOOP ( 'NONE', ( #12363, #10591, #6766, #20592 ) ) ;
#16158=DIRECTION ( 'NONE',  ( -0.7071067811865474617, 0.000000000000000000, -0.7071067811865474617 ) ) ;
#16163=CARTESIAN_POINT ( 'NONE',  ( 0.000000000000000000, 9.000000000000001776, 1.000000000000000000 ) ) ;
#16169=CARTESIAN_POINT ( 'NONE',  ( -15.11404127825609223, 4.999999999999999112, 0.000000000000000000 ) ) ;
#16176=VERTEX_POINT ( 'NONE', #17566 ) ;
#16179=VERTEX_POINT ( 'NONE', #3345 ) ;
#16180=VERTEX_POINT ( 'NONE', #3240 ) ;
#16181=DIRECTION ( 'NONE',  ( 0.000000000000000000, 1.000000000000000000, 0.000000000000000000 ) ) ;
#16184=ORIENTED_EDGE ( 'NONE', *, *, #15603, .F. ) ;
#16187=ADVANCED_FACE ( 'NONE', ( #8164 ), #9723, .T. ) ;
#16188=ADVANCED_FACE ( 'NONE', ( #14530 ), #8060, .T. ) ;
#16195=DIRECTION ( 'NONE',  ( -0.000000000000000000, -0.000000000000000000, -1.000000000000000000 ) ) ;
#16203=DIRECTION ( 'NONE',  ( -0.000000000000000000, -0.000000000000000000, -1.000000000000000000 ) ) ;
#16204=FACE_OUTER_BOUND ( 'NONE', #9563, .T. ) ;
#16205=ORIENTED_EDGE ( 'NONE', *, *, #17813, .T. ) ;
#16219=PLANE ( 'NONE',  #12723 ) ;
#16222=ADVANCED_FACE ( 'NONE', ( #5120 ), #8365, .T. ) ;
#16229=DIRECTION ( 'NONE',  ( 0.000000000000000000, 0.000000000000000000, 1.000000000000000000 ) ) ;
#16230=ORIENTED_EDGE ( 'NONE', *, *, #1822, .T. ) ;
#16231=ORIENTED_EDGE ( 'NONE', *, *, #18634, .F. ) ;
#16253=EDGE_LOOP ( 'NONE', ( #11085, #12466, #4341, #11274 ) ) ;
#16254=FACE_OUTER_BOUND ( 'NONE', #9655, .T. ) ;
#16255=CARTESIAN_POINT ( 'NONE',  ( -27.49999999999999645, -4.770489558936219510E-14, 1.000000000000000000 ) ) ;
#16260=LINE ( 'NONE', #15097, #9389 ) ;
#16261=CARTESIAN_POINT ( 'NONE',  ( 0.000000000000000000, 4.999999999999999112, 0.000000000000000000 ) ) ;
#16262=CARTESIAN_POINT ( 'NONE',  ( 0.000000000000000000, 0.000000000000000000, 9.999999999999998224 ) ) ;
#16263=DIRECTION ( 'NONE',  ( 0.000000000000000000, 1.000000000000000000, 0.000000000000000000 ) ) ;
#16274=ORIENTED_EDGE ( 'NONE', *, *, #4276, .F. ) ;
#16277=ORIENTED_EDGE ( 'NONE', *, *, #10784, .F. ) ;
#16280=ORIENTED_EDGE ( 'NONE', *, *, #20472, .T. ) ;
#16289=LINE ( 'NONE', #14719, #12196 ) ;
#16291=ORIENTED_EDGE ( 'NONE', *, *, #17030, .T. ) ;
#16306=CARTESIAN_POINT ( 'NONE',  ( 15.36404127825609400, 9.000000000000001776, 1.000000000000000000 ) ) ;
#16307=DIRECTION ( 'NONE',  ( -0.000000000000000000, 0.000000000000000000, 1.000000000000000000 ) ) ;
#16315=LINE ( 'NONE', #17988, #13730 ) ;
#16322=VERTEX_POINT ( 'NONE', #15042 ) ;
#16325=CARTESIAN_POINT ( 'NONE',  ( -5.433390479346035029, 0.000000000000000000, 1.000000000000000000 ) ) ;
#16327=VERTEX_POINT ( 'NONE', #826 ) ;
#16328=CARTESIAN_POINT ( 'NONE',  ( -7.869520639128047002, 4.999999999999999112, 1.000000000000000000 ) ) ;
#16350=VERTEX_POINT ( 'NONE', #5217 ) ;
#16351=VECTOR ( 'NONE', #14570, 1000.000000000000000 ) ;
#16352=EDGE_LOOP ( 'NONE', ( #5338, #11187, #9222, #9818 ) ) ;
#16361=EDGE_CURVE ( 'NONE', #3716, #11889, #17138, .T. ) ;
#16366=EDGE_LOOP ( 'NONE', ( #20047, #6884, #1061, #12278 ) ) ;
#16371=VERTEX_POINT ( 'NONE', #19660 ) ;
#16373=PLANE ( 'NONE',  #14373 ) ;
#16374=ORIENTED_EDGE ( 'NONE', *, *, #17838, .F. ) ;
#16377=VERTEX_POINT ( 'NONE', #2488 ) ;
#16379=AXIS2_PLACEMENT_3D ( 'NONE', #1142, #4169, #2281 ) ;
#16384=LINE ( 'NONE', #8754, #10316 ) ;
#16385=LINE ( 'NONE', #19442, #19034 ) ;
#16388=PLANE ( 'NONE',  #613 ) ;
#16394=EDGE_CURVE ( 'NONE', #6239, #13354, #13474, .T. ) ;
#16400=VECTOR ( 'NONE', #18775, 1000.000000000000000 ) ;
#16401=CARTESIAN_POINT ( 'NONE',  ( -20.00000000000000000, 0.000000000000000000, 2.000000000000000000 ) ) ;
#16402=FACE_OUTER_BOUND ( 'NONE', #11998, .T. ) ;
#16403=VECTOR ( 'NONE', #12347, 1000.000000000000000 ) ;
#16405=ORIENTED_EDGE ( 'NONE', *, *, #4350, .T. ) ;
#16409=CARTESIAN_POINT ( 'NONE',  ( 0.000000000000000000, 0.000000000000000000, 1.000000000000000000 ) ) ;
#16411=VECTOR ( 'NONE', #13505, 1000.000000000000000 ) ;
#16422=ORIENTED_EDGE ( 'NONE', *, *, #5438, .F. ) ;
#16423=ORIENTED_EDGE ( 'NONE', *, *, #7078, .T. ) ;
#16425=DIRECTION ( 'NONE',  ( -0.000000000000000000, -0.000000000000000000, -1.000000000000000000 ) ) ;
#16429=VECTOR ( 'NONE', #17240, 1000.000000000000000 ) ;
#16430=CARTESIAN_POINT ( 'NONE',  ( 0.000000000000000000, 4.999999999999999112, 1.000000000000000000 ) ) ;
#16431=CARTESIAN_POINT ( 'NONE',  ( -22.85856191738413656, 9.000000000000001776, 1.000000000000000000 ) ) ;
#16432=CARTESIAN_POINT ( 'NONE',  ( 0.000000000000000000, 9.000000000000001776, 1.000000000000000000 ) ) ;
#16434=DIRECTION ( 'NONE',  ( 0.000000000000000000, -0.000000000000000000, 1.000000000000000000 ) ) ;
#16436=EDGE_CURVE ( 'NONE', #14361, #4739, #3956, .T. ) ;
#16437=EDGE_CURVE ( 'NONE', #5735, #18810, #15664, .T. ) ;
#16443=VECTOR ( 'NONE', #3726, 1000.000000000000000 ) ;
#16449=VERTEX_POINT ( 'NONE', #15354 ) ;
#16460=DIRECTION ( 'NONE',  ( -0.000000000000000000, -0.000000000000000000, -1.000000000000000000 ) ) ;
#16469=VERTEX_POINT ( 'NONE', #17132 ) ;
#16477=ORIENTED_EDGE ( 'NONE', *, *, #19502, .F. ) ;
#16492=DIRECTION ( 'NONE',  ( 0.000000000000000000, -1.000000000000000000, 0.000000000000000000 ) ) ;
#16495=VERTEX_POINT ( 'NONE', #18606 ) ;
#16501=ORIENTED_EDGE ( 'NONE', *, *, #14375, .T. ) ;
#16503=EDGE_CURVE ( 'NONE', #16571, #15008, #20501, .T. ) ;
#16508=ADVANCED_FACE ( 'NONE', ( #2593 ), #20286, .T. ) ;
#16512=EDGE_CURVE ( 'NONE', #9049, #10249, #5747, .T. ) ;
#16514=DIRECTION ( 'NONE',  ( 0.000000000000000000, -1.000000000000000000, 0.000000000000000000 ) ) ;
#16522=ORIENTED_EDGE ( 'NONE', *, *, #7502, .F. ) ;
#16529=DIRECTION ( 'NONE',  ( -1.000000000000000000, 0.000000000000000000, 0.000000000000000000 ) ) ;
#16530=CARTESIAN_POINT ( 'NONE',  ( 23.60856191738414012, 9.000000000000001776, 0.000000000000000000 ) ) ;
#16532=PLANE ( 'NONE',  #8530 ) ;
#16534=DIRECTION ( 'NONE',  ( 0.000000000000000000, 1.000000000000000000, -0.000000000000000000 ) ) ;
#16535=VECTOR ( 'NONE', #4597, 1000.000000000000000 ) ;
#16544=ORIENTED_EDGE ( 'NONE', *, *, #11586, .T. ) ;
#16548=ORIENTED_EDGE ( 'NONE', *, *, #18430, .T. ) ;
#16549=EDGE_CURVE ( 'NONE', #6959, #17483, #8980, .T. ) ;
#16551=EDGE_CURVE ( 'NONE', #14519, #4780, #13673, .T. ) ;
#16552=CARTESIAN_POINT ( 'NONE',  ( -26.04469207716615031, 9.000000000000001776, 1.000000000000000000 ) ) ;
#16554=CARTESIAN_POINT ( 'NONE',  ( -26.04469207716614321, -2.255140518769849223E-14, 1.000000000000000000 ) ) ;
#16570=ORIENTED_EDGE ( 'NONE', *, *, #20354, .T. ) ;
#16571=VERTEX_POINT ( 'NONE', #6157 ) ;
#16575=ORIENTED_EDGE ( 'NONE', *, *, #17670, .F. ) ;
#16581=EDGE_CURVE ( 'NONE', #12176, #17531, #7617, .T. ) ;
#16591=VERTEX_POINT ( 'NONE', #12424 ) ;
#16593=DIRECTION ( 'NONE',  ( 1.000000000000000000, 0.000000000000000000, -0.000000000000000000 ) ) ;
#16595=ORIENTED_EDGE ( 'NONE', *, *, #18999, .T. ) ;
#16602=DIRECTION ( 'NONE',  ( 0.000000000000000000, 0.000000000000000000, 1.000000000000000000 ) ) ;
#16603=DIRECTION ( 'NONE',  ( -0.000000000000000000, -0.000000000000000000, -1.000000000000000000 ) ) ;
#16609=ORIENTED_EDGE ( 'NONE', *, *, #17838, .T. ) ;
#16610=CARTESIAN_POINT ( 'NONE',  ( 4.999999999999998224, 0.000000000000000000, 9.999999999999998224 ) ) ;
#16615=ORIENTED_EDGE ( 'NONE', *, *, #19788, .T. ) ;
#16617=EDGE_CURVE ( 'NONE', #5681, #13158, #18714, .T. ) ;
#16623=CARTESIAN_POINT ( 'NONE',  ( -9.805650798910056309, 0.000000000000000000, 0.000000000000000000 ) ) ;
#16624=DIRECTION ( 'NONE',  ( -0.000000000000000000, -0.000000000000000000, -1.000000000000000000 ) ) ;
#16626=DIRECTION ( 'NONE',  ( 1.000000000000000000, 0.000000000000000000, -0.000000000000000000 ) ) ;
#16647=EDGE_LOOP ( 'NONE', ( #3723, #1875, #18569, #6511 ) ) ;
#16650=CIRCLE ( 'NONE', #7646, 2.999999999999999112 ) ;
#16657=DIRECTION ( 'NONE',  ( 0.000000000000000000, -0.000000000000000000, 1.000000000000000000 ) ) ;
#16660=DIRECTION ( 'NONE',  ( 1.000000000000000000, 0.000000000000000000, 0.000000000000000000 ) ) ;
#16664=VECTOR ( 'NONE', #19204, 1000.000000000000000 ) ;
#16671=VECTOR ( 'NONE', #3639, 1000.000000000000000 ) ;
#16675=ORIENTED_EDGE ( 'NONE', *, *, #10818, .F. ) ;
#16676=VERTEX_POINT ( 'NONE', #20597 ) ;
#16677=LINE ( 'NONE', #7073, #6377 ) ;
#16681=ORIENTED_EDGE ( 'NONE', *, *, #7052, .T. ) ;
#16703=DIRECTION ( 'NONE',  ( -0.8660254037844417052, 0.4999999999999948375, 0.000000000000000000 ) ) ;
#16704=( GEOMETRIC_REPRESENTATION_CONTEXT ( 3 ) GLOBAL_UNCERTAINTY_ASSIGNED_CONTEXT ( ( #7769 ) ) GLOBAL_UNIT_ASSIGNED_CONTEXT ( ( #18732, #10981, #9305 ) ) REPRESENTATION_CONTEXT ( 'NONE', 'WORKASPACE' ) );
#16706=ORIENTED_EDGE ( 'NONE', *, *, #8129, .F. ) ;
#16708=AXIS2_PLACEMENT_3D ( 'NONE', #3780, #16529, #2205 ) ;
#16711=CARTESIAN_POINT ( 'NONE',  ( -18.98630159782011262, 4.999999999999999112, 1.000000000000000000 ) ) ;
#16713=LINE ( 'NONE', #8781, #10033 ) ;
#16715=DIRECTION ( 'NONE',  ( 0.000000000000000000, 1.000000000000000000, -0.000000000000000000 ) ) ;
#16738=LINE ( 'NONE', #945, #7121 ) ;
#16743=AXIS2_PLACEMENT_3D ( 'NONE', #11360, #16181, #17749 ) ;
#16744=DIRECTION ( 'NONE',  ( 0.000000000000000000, 1.000000000000000000, 0.000000000000000000 ) ) ;
#16751=CARTESIAN_POINT ( 'NONE',  ( 3.999999999999999112, -7.500000000000047073, 2.000000000000000000 ) ) ;
#16753=VECTOR ( 'NONE', #9835, 1000.000000000000000 ) ;
#16763=EDGE_CURVE ( 'NONE', #13679, #3772, #18270, .T. ) ;
#16766=CIRCLE ( 'NONE', #4415, 0.5000000000000000000 ) ;
#16770=DIRECTION ( 'NONE',  ( 0.000000000000000000, 1.000000000000000000, 0.000000000000000000 ) ) ;
#16776=EDGE_LOOP ( 'NONE', ( #1711, #19629, #2748, #480 ) ) ;
#16782=ORIENTED_EDGE ( 'NONE', *, *, #11787, .F. ) ;
#16784=CARTESIAN_POINT ( 'NONE',  ( 0.000000000000000000, 9.000000000000001776, 1.000000000000000000 ) ) ;
#16785=ORIENTED_EDGE ( 'NONE', *, *, #9030, .F. ) ;
#16786=ORIENTED_EDGE ( 'NONE', *, *, #3216, .T. ) ;
#16787=VECTOR ( 'NONE', #14550, 1000.000000000000000 ) ;
#16789=ORIENTED_EDGE ( 'NONE', *, *, #3761, .F. ) ;
#16795=CARTESIAN_POINT ( 'NONE',  ( -13.50000000000000178, 0.000000000000000000, 2.000000000000000000 ) ) ;
#16803=EDGE_CURVE ( 'NONE', #381, #3752, #10845, .T. ) ;
#16809=ORIENTED_EDGE ( 'NONE', *, *, #796, .F. ) ;
#16812=VECTOR ( 'NONE', #7943, 1000.000000000000000 ) ;
#16813=ORIENTED_EDGE ( 'NONE', *, *, #17219, .F. ) ;
#16823=FACE_OUTER_BOUND ( 'NONE', #18335, .T. ) ;
#16824=DIRECTION ( 'NONE',  ( -1.000000000000000000, 0.000000000000000000, 0.000000000000000000 ) ) ;
#16831=LINE ( 'NONE', #12531, #8093 ) ;
#16835=ORIENTED_EDGE ( 'NONE', *, *, #18173, .F. ) ;
#16841=CARTESIAN_POINT ( 'NONE',  ( -5.933390479346035029, 4.999999999999999112, 1.000000000000000000 ) ) ;
#16842=LINE ( 'NONE', #10364, #17382 ) ;
#16848=CARTESIAN_POINT ( 'NONE',  ( 13.42791111847407848, 4.999999999999999112, 0.000000000000000000 ) ) ;
#16862=VERTEX_POINT ( 'NONE', #4460 ) ;
#16863=DIRECTION ( 'NONE',  ( 0.000000000000000000, -0.000000000000000000, 1.000000000000000000 ) ) ;
#16865=DIRECTION ( 'NONE',  ( -0.000000000000000000, -0.000000000000000000, -1.000000000000000000 ) ) ;
#16870=DIRECTION ( 'NONE',  ( 0.000000000000000000, -1.000000000000000000, 0.000000000000000000 ) ) ;
#16871=VECTOR ( 'NONE', #14371, 1000.000000000000000 ) ;
#16875=ORIENTED_EDGE ( 'NONE', *, *, #17638, .T. ) ;
#16877=CARTESIAN_POINT ( 'NONE',  ( -5.999999999999999112, -2.500000000000047518, 9.999999999999998224 ) ) ;
#16886=ORIENTED_EDGE ( 'NONE', *, *, #17706, .F. ) ;
#16894=CARTESIAN_POINT ( 'NONE',  ( 0.000000000000000000, 9.000000000000001776, 1.000000000000000000 ) ) ;
#16900=CARTESIAN_POINT ( 'NONE',  ( -13.17791111847408025, 0.000000000000000000, 1.000000000000000000 ) ) ;
#16904=EDGE_CURVE ( 'NONE', #19089, #6994, #8952, .T. ) ;
#16906=ORIENTED_EDGE ( 'NONE', *, *, #14634, .T. ) ;
#16909=VERTEX_POINT ( 'NONE', #12091 ) ;
#16910=PLANE ( 'NONE',  #17287 ) ;
#16914=VECTOR ( 'NONE', #8209, 1000.000000000000000 ) ;
#16915=EDGE_LOOP ( 'NONE', ( #5867, #11364, #18667, #811 ) ) ;
#16921=CARTESIAN_POINT ( 'NONE',  ( 0.000000000000000000, 0.000000000000000000, 1.000000000000000000 ) ) ;
#16927=ORIENTED_EDGE ( 'NONE', *, *, #20290, .T. ) ;
#16928=EDGE_CURVE ( 'NONE', #19095, #49, #1005, .T. ) ;
#16930=CARTESIAN_POINT ( 'NONE',  ( 21.67243175760212637, 4.999999999999999112, 0.000000000000000000 ) ) ;
#16939=LINE ( 'NONE', #5656, #10810 ) ;
#16943=DIRECTION ( 'NONE',  ( 0.000000000000000000, -0.000000000000000000, 1.000000000000000000 ) ) ;
#16951=DIRECTION ( 'NONE',  ( 1.000000000000000000, 0.000000000000000000, 0.000000000000000000 ) ) ;
#16959=VECTOR ( 'NONE', #10020, 1000.000000000000000 ) ;
#16962=ORIENTED_EDGE ( 'NONE', *, *, #7798, .F. ) ;
#16970=DIRECTION ( 'NONE',  ( 1.000000000000000000, 0.000000000000000000, 0.000000000000000000 ) ) ;
#16972=VECTOR ( 'NONE', #17233, 1000.000000000000000 ) ;
#16977=EDGE_LOOP ( 'NONE', ( #19604, #9510, #943, #11339 ) ) ;
#16987=ORIENTED_EDGE ( 'NONE', *, *, #3709, .T. ) ;
#16992=AXIS2_PLACEMENT_3D ( 'NONE', #2589, #12214, #918 ) ;
#16995=DIRECTION ( 'NONE',  ( -0.000000000000000000, -0.000000000000000000, -1.000000000000000000 ) ) ;
#16999=LINE ( 'NONE', #7283, #4316 ) ;
#17002=DIRECTION ( 'NONE',  ( -1.000000000000000000, 0.000000000000000000, -0.000000000000000000 ) ) ;
#17003=VECTOR ( 'NONE', #12535, 1000.000000000000000 ) ;
#17004=DIRECTION ( 'NONE',  ( 1.000000000000000000, 0.000000000000000000, 0.000000000000000000 ) ) ;
#17005=LINE ( 'NONE', #5725, #15383 ) ;
#17006=CARTESIAN_POINT ( 'NONE',  ( 8.119520639128047890, 4.999999999999999112, 1.000000000000000000 ) ) ;
#17016=CARTESIAN_POINT ( 'NONE',  ( 19.23630159782011617, 0.000000000000000000, 1.000000000000000000 ) ) ;
#17019=VECTOR ( 'NONE', #7249, 1000.000000000000000 ) ;
#17024=EDGE_CURVE ( 'NONE', #17249, #2461, #13647, .T. ) ;
#17027=DIRECTION ( 'NONE',  ( 0.000000000000000000, 1.000000000000000000, -0.000000000000000000 ) ) ;
#17029=ADVANCED_FACE ( 'NONE', ( #20160 ), #17307, .T. ) ;
#17030=EDGE_CURVE ( 'NONE', #5395, #20292, #58, .T. ) ;
#17035=EDGE_LOOP ( 'NONE', ( #8797, #19818, #9581, #1353 ) ) ;
#17039=VECTOR ( 'NONE', #16660, 1000.000000000000000 ) ;
#17042=VERTEX_POINT ( 'NONE', #6443 ) ;
#17043=VERTEX_POINT ( 'NONE', #11240 ) ;
#17045=DIRECTION ( 'NONE',  ( 0.000000000000000000, -0.000000000000000000, 1.000000000000000000 ) ) ;
#17049=ORIENTED_EDGE ( 'NONE', *, *, #17412, .F. ) ;
#17052=EDGE_CURVE ( 'NONE', #5289, #4330, #14480, .T. ) ;
#17054=CARTESIAN_POINT ( 'NONE',  ( 15.86404127825609400, 4.999999999999999112, 1.000000000000000000 ) ) ;
#17056=VECTOR ( 'NONE', #2656, 1000.000000000000000 ) ;
#17061=DIRECTION ( 'NONE',  ( -0.000000000000000000, -0.000000000000000000, -1.000000000000000000 ) ) ;
#17067=VECTOR ( 'NONE', #3054, 1000.000000000000000 ) ;
#17068=DIRECTION ( 'NONE',  ( 0.000000000000000000, 1.000000000000000000, -0.000000000000000000 ) ) ;
#17071=VECTOR ( 'NONE', #10498, 1000.000000000000114 ) ;
#17080=PLANE ( 'NONE',  #11543 ) ;
#17081=CARTESIAN_POINT ( 'NONE',  ( 4.999999999999998224, 0.000000000000000000, 9.999999999999998224 ) ) ;
#17082=DIRECTION ( 'NONE',  ( -1.000000000000000000, 0.000000000000000000, 0.000000000000000000 ) ) ;
#17083=VECTOR ( 'NONE', #11177, 1000.000000000000000 ) ;
#17090=ADVANCED_FACE ( 'NONE', ( #12808 ), #19206, .T. ) ;
#17097=ORIENTED_EDGE ( 'NONE', *, *, #8645, .F. ) ;
#17119=ORIENTED_EDGE ( 'NONE', *, *, #3786, .T. ) ;
#17124=EDGE_LOOP ( 'NONE', ( #13155, #15617, #657, #3519 ) ) ;
#17126=ORIENTED_EDGE ( 'NONE', *, *, #18622, .T. ) ;
#17127=FACE_OUTER_BOUND ( 'NONE', #19014, .T. ) ;
#17128=VECTOR ( 'NONE', #8303, 1000.000000000000000 ) ;
#17132=CARTESIAN_POINT ( 'NONE',  ( 3.999999999999999112, -2.500000000000047518, 2.000000000000000000 ) ) ;
#17134=LINE ( 'NONE', #7902, #20391 ) ;
#17138=CIRCLE ( 'NONE', #8134, 0.4999999999999987232 ) ;
#17141=CARTESIAN_POINT ( 'NONE',  ( 27.50000000000000355, 3.000000000000000888, 1.000000000000000000 ) ) ;
#17144=VECTOR ( 'NONE', #3338, 1000.000000000000000 ) ;
#17145=EDGE_CURVE ( 'NONE', #16377, #431, #17618, .T. ) ;
#17147=CARTESIAN_POINT ( 'NONE',  ( 0.000000000000000000, 9.000000000000001776, 1.000000000000000000 ) ) ;
#17148=ORIENTED_EDGE ( 'NONE', *, *, #17052, .T. ) ;
#17151=CARTESIAN_POINT ( 'NONE',  ( 17.80017143803810242, 4.999999999999999112, 1.000000000000000000 ) ) ;
#17153=DIRECTION ( 'NONE',  ( 1.000000000000000000, 0.000000000000000000, 0.000000000000000000 ) ) ;
#17155=ORIENTED_EDGE ( 'NONE', *, *, #8111, .T. ) ;
#17159=LINE ( 'NONE', #10576, #16535 ) ;
#17182=DIRECTION ( 'NONE',  ( 1.000000000000000000, 0.000000000000000000, 0.000000000000000000 ) ) ;
#17184=CARTESIAN_POINT ( 'NONE',  ( 17.80017143803810242, 0.000000000000000000, 0.000000000000000000 ) ) ;
#17197=VERTEX_POINT ( 'NONE', #19414 ) ;
#17198=VERTEX_POINT ( 'NONE', #11046 ) ;
#17204=LINE ( 'NONE', #2881, #9526 ) ;
#17212=CARTESIAN_POINT ( 'NONE',  ( 0.000000000000000000, 9.000000000000001776, 1.000000000000000000 ) ) ;
#17219=EDGE_CURVE ( 'NONE', #734, #20304, #2991, .T. ) ;
#17221=DIRECTION ( 'NONE',  ( -0.000000000000000000, -0.000000000000000000, -1.000000000000000000 ) ) ;
#17227=VERTEX_POINT ( 'NONE', #14167 ) ;
#17229=EDGE_CURVE ( 'NONE', #17871, #10048, #17420, .T. ) ;
#17232=DIRECTION ( 'NONE',  ( 1.000000000000000000, 0.000000000000000000, 0.000000000000000000 ) ) ;
#17233=DIRECTION ( 'NONE',  ( 0.000000000000000000, -1.000000000000000000, 0.000000000000000000 ) ) ;
#17234=CARTESIAN_POINT ( 'NONE',  ( -27.50000000000000355, 3.000000000000000888, 1.000000000000000000 ) ) ;
#17238=ORIENTED_EDGE ( 'NONE', *, *, #15162, .T. ) ;
#17240=DIRECTION ( 'NONE',  ( 0.000000000000000000, 1.000000000000000000, -0.000000000000000000 ) ) ;
#17243=DIRECTION ( 'NONE',  ( 1.000000000000000000, 0.000000000000000000, 0.000000000000000000 ) ) ;
#17246=CARTESIAN_POINT ( 'NONE',  ( -13.50000000000000178, -0.4999999999999987232, 1.000000000000000000 ) ) ;
#17247=VERTEX_POINT ( 'NONE', #15842 ) ;
#17248=CARTESIAN_POINT ( 'NONE',  ( 23.10856191738414012, 9.000000000000001776, 1.000000000000000000 ) ) ;
#17249=VERTEX_POINT ( 'NONE', #7900 ) ;
#17252=LINE ( 'NONE', #5970, #9201 ) ;
#17266=CIRCLE ( 'NONE', #3255, 0.5000000000000000000 ) ;
#17274=ADVANCED_FACE ( 'NONE', ( #13315 ), #7160, .T. ) ;
#17276=DIRECTION ( 'NONE',  ( 1.000000000000000000, 0.000000000000000000, 0.000000000000000000 ) ) ;
#17277=LINE ( 'NONE', #3268, #15 ) ;
#17284=EDGE_CURVE ( 'NONE', #19147, #15669, #6943, .T. ) ;
#17286=CARTESIAN_POINT ( 'NONE',  ( -13.00000000000000355, 6.123233995736752477E-17, 2.000000000000000000 ) ) ;
#17287=AXIS2_PLACEMENT_3D ( 'NONE', #8658, #12107, #15340 ) ;
#17292=FACE_OUTER_BOUND ( 'NONE', #20381, .T. ) ;
#17297=EDGE_LOOP ( 'NONE', ( #6428, #17536, #14250, #6691 ) ) ;
#17304=EDGE_CURVE ( 'NONE', #11462, #15883, #469, .T. ) ;
#17307=PLANE ( 'NONE',  #6528 ) ;
#17310=CARTESIAN_POINT ( 'NONE',  ( -2.981555974335140152E-16, 2.500000000000002220, 1.500000000000000000 ) ) ;
#17319=DIRECTION ( 'NONE',  ( -0.000000000000000000, -0.000000000000000000, -1.000000000000000000 ) ) ;
#17328=EDGE_LOOP ( 'NONE', ( #1946, #9529, #3232, #18545 ) ) ;
#17332=VECTOR ( 'NONE', #20514, 1000.000000000000000 ) ;
#17333=EDGE_CURVE ( 'NONE', #11889, #6051, #16260, .T. ) ;
#17337=VECTOR ( 'NONE', #11167, 1000.000000000000000 ) ;
#17344=CARTESIAN_POINT ( 'NONE',  ( -13.50000000000000178, 0.000000000000000000, 2.000000000000000000 ) ) ;
#17347=VERTEX_POINT ( 'NONE', #10287 ) ;
#17348=ADVANCED_FACE ( 'NONE', ( #3705 ), #19716, .F. ) ;
#17351=ORIENTED_EDGE ( 'NONE', *, *, #970, .F. ) ;
#17352=DIRECTION ( 'NONE',  ( -0.000000000000000000, -0.000000000000000000, -1.000000000000000000 ) ) ;
#17353=( LENGTH_UNIT ( ) NAMED_UNIT ( * ) SI_UNIT ( .MILLI., .METRE. ) );
#17362=CARTESIAN_POINT ( 'NONE',  ( 0.000000000000000000, -0.5000000000000004441, 1.000000000000000000 ) ) ;
#17367=LINE ( 'NONE', #9428, #18754 ) ;
#17372=ORIENTED_EDGE ( 'NONE', *, *, #12067, .T. ) ;
#17377=AXIS2_PLACEMENT_3D ( 'NONE', #16921, #2706, #4170 ) ;
#17380=CARTESIAN_POINT ( 'NONE',  ( 0.000000000000000000, 4.999999999999999112, 1.000000000000000000 ) ) ;
#17382=VECTOR ( 'NONE', #19681, 1000.000000000000000 ) ;
#17395=VECTOR ( 'NONE', #6213, 1000.000000000000000 ) ;
#17405=CARTESIAN_POINT ( 'NONE',  ( 23.60856191738414012, 0.000000000000000000, 1.000000000000000000 ) ) ;
#17408=ORIENTED_EDGE ( 'NONE', *, *, #8949, .F. ) ;
#17409=DIRECTION ( 'NONE',  ( 1.000000000000000000, 0.000000000000000000, 0.000000000000000000 ) ) ;
#17412=EDGE_CURVE ( 'NONE', #3772, #3612, #8517, .T. ) ;
#17413=EDGE_LOOP ( 'NONE', ( #13025, #18089, #12715, #3413 ) ) ;
#17416=AXIS2_PLACEMENT_3D ( 'NONE', #18971, #8091, #9339 ) ;
#17417=AXIS2_PLACEMENT_3D ( 'NONE', #18160, #1109, #5600 ) ;
#17420=LINE ( 'NONE', #3096, #12518 ) ;
#17422=DIRECTION ( 'NONE',  ( 0.000000000000000000, -0.000000000000000000, 1.000000000000000000 ) ) ;
#17431=CARTESIAN_POINT ( 'NONE',  ( -3.999999999999999112, -2.500000000000047518, 9.999999999999998224 ) ) ;
#17439=CARTESIAN_POINT ( 'NONE',  ( 0.000000000000000000, 4.999999999999999112, 0.000000000000000000 ) ) ;
#17449=ORIENTED_EDGE ( 'NONE', *, *, #19098, .T. ) ;
#17456=DIRECTION ( 'NONE',  ( -0.000000000000000000, 0.000000000000000000, 1.000000000000000000 ) ) ;
#17458=VERTEX_POINT ( 'NONE', #11853 ) ;
#17460=ORIENTED_EDGE ( 'NONE', *, *, #4276, .T. ) ;
#17463=CARTESIAN_POINT ( 'NONE',  ( 19.73630159782011617, 9.000000000000001776, 1.000000000000000000 ) ) ;
#17467=LINE ( 'NONE', #11500, #1145 ) ;
#17483=VERTEX_POINT ( 'NONE', #9036 ) ;
#17495=ORIENTED_EDGE ( 'NONE', *, *, #11235, .T. ) ;
#17497=DIRECTION ( 'NONE',  ( -0.000000000000000000, -0.000000000000000000, -1.000000000000000000 ) ) ;
#17503=DIRECTION ( 'NONE',  ( 0.000000000000000000, 0.000000000000000000, 1.000000000000000000 ) ) ;
#17507=CARTESIAN_POINT ( 'NONE',  ( -20.00000000000000000, 3.499999999999999556, 1.000000000000000000 ) ) ;
#17511=DIRECTION ( 'NONE',  ( 0.000000000000000000, -1.000000000000000000, 0.000000000000000000 ) ) ;
#17513=CARTESIAN_POINT ( 'NONE',  ( 0.000000000000000000, 4.999999999999999112, 0.000000000000000000 ) ) ;
#17526=EDGE_CURVE ( 'NONE', #18629, #16327, #13621, .T. ) ;
#17529=ORIENTED_EDGE ( 'NONE', *, *, #11895, .F. ) ;
#17531=VERTEX_POINT ( 'NONE', #7259 ) ;
#17533=ORIENTED_EDGE ( 'NONE', *, *, #13403, .F. ) ;
#17534=PLANE ( 'NONE',  #19135 ) ;
#17536=ORIENTED_EDGE ( 'NONE', *, *, #1802, .F. ) ;
#17537=CARTESIAN_POINT ( 'NONE',  ( 0.000000000000000000, 9.000000000000001776, 0.000000000000000000 ) ) ;
#17554=EDGE_CURVE ( 'NONE', #20304, #510, #13729, .T. ) ;
#17566=CARTESIAN_POINT ( 'NONE',  ( 13.92791111847407848, 9.000000000000001776, 0.000000000000000000 ) ) ;
#17568=EDGE_CURVE ( 'NONE', #15008, #7330, #5795, .T. ) ;
#17569=EDGE_CURVE ( 'NONE', #20470, #4209, #12165, .T. ) ;
#17582=ORIENTED_EDGE ( 'NONE', *, *, #14329, .T. ) ;
#17583=ADVANCED_FACE ( 'NONE', ( #5582 ), #13830, .T. ) ;
#17585=DIRECTION ( 'NONE',  ( -0.000000000000000000, -0.000000000000000000, -1.000000000000000000 ) ) ;
#17587=LINE ( 'NONE', #8083, #357 ) ;
#17591=EDGE_CURVE ( 'NONE', #7736, #487, #20234, .T. ) ;
#17592=EDGE_CURVE ( 'NONE', #13818, #17197, #4325, .T. ) ;
#17595=CARTESIAN_POINT ( 'NONE',  ( 0.000000000000000000, 4.999999999999999112, 0.000000000000000000 ) ) ;
#17608=PLANE ( 'NONE',  #7009 ) ;
#17609=ORIENTED_EDGE ( 'NONE', *, *, #6410, .T. ) ;
#17611=ORIENTED_EDGE ( 'NONE', *, *, #2751, .F. ) ;
#17614=AXIS2_PLACEMENT_3D ( 'NONE', #6515, #12877, #20638 ) ;
#17618=LINE ( 'NONE', #6226, #16871 ) ;
#17620=CARTESIAN_POINT ( 'NONE',  ( 0.000000000000000000, 9.000000000000001776, 1.000000000000000000 ) ) ;
#17621=CARTESIAN_POINT ( 'NONE',  ( 20.00000000000000000, 2.500000000000004885, 1.500000000000000000 ) ) ;
#17622=CARTESIAN_POINT ( 'NONE',  ( 0.3749999999999968914, 0.000000000000000000, 0.000000000000000000 ) ) ;
#17623=LINE ( 'NONE', #3099, #9712 ) ;
#17632=VECTOR ( 'NONE', #4907, 1000.000000000000000 ) ;
#17635=ORIENTED_EDGE ( 'NONE', *, *, #10759, .F. ) ;
#17636=CARTESIAN_POINT ( 'NONE',  ( -21.42243175760212637, 4.999999999999999112, 0.000000000000000000 ) ) ;
#17638=EDGE_CURVE ( 'NONE', #18591, #11254, #20333, .T. ) ;
#17645=AXIS2_PLACEMENT_3D ( 'NONE', #18433, #1451, #5560 ) ;
#17649=VECTOR ( 'NONE', #4475, 1000.000000000000000 ) ;
#17657=DIRECTION ( 'NONE',  ( 0.000000000000000000, -0.000000000000000000, 1.000000000000000000 ) ) ;
#17662=VERTEX_POINT ( 'NONE', #1290 ) ;
#17666=AXIS2_PLACEMENT_3D ( 'NONE', #8877, #4264, #18504 ) ;
#17670=EDGE_CURVE ( 'NONE', #2072, #12804, #14040, .T. ) ;
#17673=EDGE_CURVE ( 'NONE', #8680, #9082, #6107, .T. ) ;
#17676=DIRECTION ( 'NONE',  ( -0.000000000000000000, 0.000000000000000000, -1.000000000000000000 ) ) ;
#17682=FACE_OUTER_BOUND ( 'NONE', #10505, .T. ) ;
#17688=ORIENTED_EDGE ( 'NONE', *, *, #9878, .F. ) ;
#17694=CARTESIAN_POINT ( 'NONE',  ( 21.17243175760212637, 9.000000000000001776, 0.000000000000000000 ) ) ;
#17695=FACE_BOUND ( 'NONE', #460, .T. ) ;
#17700=VECTOR ( 'NONE', #6333, 1000.000000000000000 ) ;
#17704=CARTESIAN_POINT ( 'NONE',  ( 0.000000000000000000, 4.999999999999999112, 0.000000000000000000 ) ) ;
#17706=EDGE_CURVE ( 'NONE', #3209, #20155, #17277, .T. ) ;
#17709=ORIENTED_EDGE ( 'NONE', *, *, #8721, .T. ) ;
#17722=EDGE_CURVE ( 'NONE', #3444, #3944, #1706, .T. ) ;
#17723=EDGE_LOOP ( 'NONE', ( #12076, #16205 ) ) ;
#17724=EDGE_CURVE ( 'NONE', #14584, #13134, #9644, .T. ) ;
#17725=CARTESIAN_POINT ( 'NONE',  ( 0.000000000000000000, 4.999999999999999112, 0.000000000000000000 ) ) ;
#17732=CARTESIAN_POINT ( 'NONE',  ( -17.11324865405191176, -11.00000000000000000, 2.000000000000000000 ) ) ;
#17736=DIRECTION ( 'NONE',  ( 0.1736481776669295540, 0.9848077530122082424, 0.000000000000000000 ) ) ;
#17737=DIRECTION ( 'NONE',  ( 0.000000000000000000, -1.000000000000000000, 0.000000000000000000 ) ) ;
#17744=EDGE_LOOP ( 'NONE', ( #7175, #506, #6855, #2321 ) ) ;
#17748=ORIENTED_EDGE ( 'NONE', *, *, #19226, .T. ) ;
#17749=DIRECTION ( 'NONE',  ( 0.000000000000000000, -0.000000000000000000, 1.000000000000000000 ) ) ;
#17751=FACE_OUTER_BOUND ( 'NONE', #3871, .T. ) ;
#17759=EDGE_CURVE ( 'NONE', #17197, #4851, #18223, .T. ) ;
#17760=DIRECTION ( 'NONE',  ( 0.000000000000000000, 1.000000000000000000, -0.000000000000000000 ) ) ;
#17771=CARTESIAN_POINT ( 'NONE',  ( 0.000000000000000000, 9.000000000000001776, 0.000000000000000000 ) ) ;
#17779=VECTOR ( 'NONE', #4964, 1000.000000000000000 ) ;
#17781=CARTESIAN_POINT ( 'NONE',  ( 13.42791111847407848, 0.000000000000000000, 1.000000000000000000 ) ) ;
#17788=EDGE_CURVE ( 'NONE', #16070, #4697, #13400, .T. ) ;
#17794=ORIENTED_EDGE ( 'NONE', *, *, #13710, .F. ) ;
#17795=ORIENTED_EDGE ( 'NONE', *, *, #3383, .F. ) ;
#17797=EDGE_CURVE ( 'NONE', #19731, #2846, #10374, .T. ) ;
#17802=CARTESIAN_POINT ( 'NONE',  ( -19.48630159782011262, 0.000000000000000000, 1.000000000000000000 ) ) ;
#17803=CARTESIAN_POINT ( 'NONE',  ( 19.23630159782011617, 4.999999999999999112, 0.000000000000000000 ) ) ;
#17813=EDGE_CURVE ( 'NONE', #11889, #3716, #18549, .T. ) ;
#17820=ORIENTED_EDGE ( 'NONE', *, *, #17973, .T. ) ;
#17823=DIRECTION ( 'NONE',  ( 1.000000000000000000, 0.000000000000000000, 0.000000000000000000 ) ) ;
#17832=DIRECTION ( 'NONE',  ( -1.000000000000000000, 0.000000000000000000, 0.000000000000000000 ) ) ;
#17833=CARTESIAN_POINT ( 'NONE',  ( 2.311130159782011972, 9.000000000000001776, 1.000000000000000000 ) ) ;
#17835=DIRECTION ( 'NONE',  ( -1.000000000000000000, 0.000000000000000000, 0.000000000000000000 ) ) ;
#17837=CARTESIAN_POINT ( 'NONE',  ( -11.24178095869206828, 0.000000000000000000, 0.000000000000000000 ) ) ;
#17838=EDGE_CURVE ( 'NONE', #3865, #16449, #7141, .T. ) ;
#17846=VECTOR ( 'NONE', #4433, 1000.000000000000000 ) ;
#17850=LINE ( 'NONE', #8230, #2731 ) ;
#17852=DIRECTION ( 'NONE',  ( -1.000000000000000000, 0.000000000000000000, 0.000000000000000000 ) ) ;
#17860=ADVANCED_FACE ( 'NONE', ( #19905 ), #12039, .T. ) ;
#17864=ORIENTED_EDGE ( 'NONE', *, *, #4167, .T. ) ;
#17870=CARTESIAN_POINT ( 'NONE',  ( -15.61404127825609223, 4.999999999999999112, 1.000000000000000000 ) ) ;
#17871=VERTEX_POINT ( 'NONE', #17234 ) ;
#17874=ADVANCED_FACE ( 'NONE', ( #854 ), #10967, .T. ) ;
#17890=VECTOR ( 'NONE', #19339, 1000.000000000000000 ) ;
#17893=VERTEX_POINT ( 'NONE', #4380 ) ;
#17898=ORIENTED_EDGE ( 'NONE', *, *, #12309, .T. ) ;
#17900=FACE_BOUND ( 'NONE', #14545, .T. ) ;
#17901=EDGE_CURVE ( 'NONE', #9026, #1111, #20598, .T. ) ;
#17905=CARTESIAN_POINT ( 'NONE',  ( -9.805650798910056309, 4.999999999999999112, 1.000000000000000000 ) ) ;
#17918=CARTESIAN_POINT ( 'NONE',  ( -26.04469207716614321, -2.255140518769849223E-14, 0.000000000000000000 ) ) ;
#17920=ORIENTED_EDGE ( 'NONE', *, *, #7098, .F. ) ;
#17921=CARTESIAN_POINT ( 'NONE',  ( 8.119520639128047890, 9.000000000000001776, 1.000000000000000000 ) ) ;
#17930=CARTESIAN_POINT ( 'NONE',  ( -11.74178095869206828, 0.000000000000000000, 0.000000000000000000 ) ) ;
#17932=DIRECTION ( 'NONE',  ( 0.000000000000000000, -0.000000000000000000, 1.000000000000000000 ) ) ;
#17946=ORIENTED_EDGE ( 'NONE', *, *, #12843, .T. ) ;
#17947=LINE ( 'NONE', #14810, #11105 ) ;
#17948=EDGE_CURVE ( 'NONE', #431, #734, #14605, .T. ) ;
#17954=DIRECTION ( 'NONE',  ( 1.000000000000000000, 0.000000000000000000, -0.000000000000000000 ) ) ;
#17961=ORIENTED_EDGE ( 'NONE', *, *, #2498, .F. ) ;
#17967=DIRECTION ( 'NONE',  ( -0.000000000000000000, -0.000000000000000000, -1.000000000000000000 ) ) ;
#17973=EDGE_CURVE ( 'NONE', #7153, #13440, #12932, .T. ) ;
#17976=EDGE_LOOP ( 'NONE', ( #6678, #5084, #4401, #5105 ) ) ;
#17977=LINE ( 'NONE', #8468, #9629 ) ;
#17983=PLANE ( 'NONE',  #9354 ) ;
#17986=EDGE_CURVE ( 'NONE', #20705, #11975, #87, .T. ) ;
#17988=CARTESIAN_POINT ( 'NONE',  ( 0.000000000000000000, 9.000000000000001776, 1.000000000000000000 ) ) ;
#17993=AXIS2_PLACEMENT_3D ( 'NONE', #8117, #9570, #19312 ) ;
#17998=LINE ( 'NONE', #8583, #11440 ) ;
#17999=EDGE_LOOP ( 'NONE', ( #14650, #13874, #8504, #5539 ) ) ;
#18001=DIRECTION ( 'NONE',  ( 0.000000000000000000, 1.000000000000000000, 0.000000000000000000 ) ) ;
#18008=AXIS2_PLACEMENT_3D ( 'NONE', #13383, #10467, #11814 ) ;
#18012=VECTOR ( 'NONE', #11976, 1000.000000000000000 ) ;
#18013=DIRECTION ( 'NONE',  ( 0.000000000000000000, 1.000000000000000000, -0.000000000000000000 ) ) ;
#18015=EDGE_CURVE ( 'NONE', #12851, #2944, #6474, .T. ) ;
#18023=DIRECTION ( 'NONE',  ( -0.000000000000000000, -0.000000000000000000, -1.000000000000000000 ) ) ;
#18024=EDGE_LOOP ( 'NONE', ( #3822, #2147, #11413, #19937 ) ) ;
#18027=ORIENTED_EDGE ( 'NONE', *, *, #11154, .T. ) ;
#18028=CARTESIAN_POINT ( 'NONE',  ( -14.00000000000000000, 0.000000000000000000, 2.000000000000000000 ) ) ;
#18030=VECTOR ( 'NONE', #16061, 1000.000000000000000 ) ;
#18036=AXIS2_PLACEMENT_3D ( 'NONE', #11216, #10138, #1491 ) ;
#18037=LINE ( 'NONE', #9879, #5718 ) ;
#18039=AXIS2_PLACEMENT_3D ( 'NONE', #1793, #16229, #8180 ) ;
#18047=AXIS2_PLACEMENT_3D ( 'NONE', #17621, #15844, #3291 ) ;
#18050=ORIENTED_EDGE ( 'NONE', *, *, #1622, .F. ) ;
#18057=CARTESIAN_POINT ( 'NONE',  ( 0.000000000000000000, 9.000000000000001776, 1.000000000000000000 ) ) ;
#18058=ADVANCED_FACE ( 'NONE', ( #19640 ), #702, .T. ) ;
#18062=AXIS2_PLACEMENT_3D ( 'NONE', #16900, #18586, #13864 ) ;
#18064=DIRECTION ( 'NONE',  ( 0.000000000000000000, -0.000000000000000000, 1.000000000000000000 ) ) ;
#18066=CARTESIAN_POINT ( 'NONE',  ( 9.555650798910054533, 9.000000000000001776, 0.000000000000000000 ) ) ;
#18067=CARTESIAN_POINT ( 'NONE',  ( 0.000000000000000000, 9.000000000000001776, 1.000000000000000000 ) ) ;
#18074=EDGE_CURVE ( 'NONE', #19969, #18591, #18273, .T. ) ;
#18081=VECTOR ( 'NONE', #670, 1000.000000000000000 ) ;
#18082=CARTESIAN_POINT ( 'NONE',  ( 21.17243175760212637, 0.000000000000000000, 1.000000000000000000 ) ) ;
#18083=DIRECTION ( 'NONE',  ( 1.000000000000000000, 0.000000000000000000, 0.000000000000000000 ) ) ;
#18089=ORIENTED_EDGE ( 'NONE', *, *, #19002, .F. ) ;
#18093=VECTOR ( 'NONE', #1348, 1000.000000000000000 ) ;
#18110=EDGE_LOOP ( 'NONE', ( #18442, #8323, #11361, #11024 ) ) ;
#18117=ADVANCED_FACE ( 'NONE', ( #11881 ), #16388, .T. ) ;
#18118=CARTESIAN_POINT ( 'NONE',  ( -3.999999999999999112, -2.500000000000047518, 7.000000000000000000 ) ) ;
#18122=DIRECTION ( 'NONE',  ( 0.000000000000000000, 1.000000000000000000, 0.000000000000000000 ) ) ;
#18127=VECTOR ( 'NONE', #4956, 1000.000000000000000 ) ;
#18132=ORIENTED_EDGE ( 'NONE', *, *, #6760, .F. ) ;
#18138=DIRECTION ( 'NONE',  ( 0.000000000000000000, -1.000000000000000000, 0.000000000000000000 ) ) ;
#18139=EDGE_CURVE ( 'NONE', #14572, #16495, #3935, .T. ) ;
#18158=ORIENTED_EDGE ( 'NONE', *, *, #15724, .F. ) ;
#18160=CARTESIAN_POINT ( 'NONE',  ( 0.000000000000000000, 9.000000000000001776, 1.000000000000000000 ) ) ;
#18161=ORIENTED_EDGE ( 'NONE', *, *, #10636, .T. ) ;
#18164=DIRECTION ( 'NONE',  ( 0.000000000000000000, 1.000000000000000000, 0.000000000000000000 ) ) ;
#18171=DIRECTION ( 'NONE',  ( 0.000000000000000000, -0.000000000000000000, 1.000000000000000000 ) ) ;
#18173=EDGE_CURVE ( 'NONE', #5029, #4594, #2162, .T. ) ;
#18183=DIRECTION ( 'NONE',  ( 0.000000000000000000, 0.000000000000000000, -1.000000000000000000 ) ) ;
#18184=EDGE_LOOP ( 'NONE', ( #12536, #14899, #17961, #16786 ) ) ;
#18192=DIRECTION ( 'NONE',  ( 1.000000000000000000, 0.000000000000000000, 0.000000000000000000 ) ) ;
#18196=CARTESIAN_POINT ( 'NONE',  ( 0.000000000000000000, 4.999999999999999112, 1.000000000000000000 ) ) ;
#18205=EDGE_CURVE ( 'NONE', #2799, #14875, #10431, .T. ) ;
#18208=EDGE_LOOP ( 'NONE', ( #11111, #13131, #8533, #5000 ) ) ;
#18209=ORIENTED_EDGE ( 'NONE', *, *, #16437, .F. ) ;
#18213=CARTESIAN_POINT ( 'NONE',  ( -4.999999999999998224, -7.500000000000047073, 9.999999999999998224 ) ) ;
#18215=CARTESIAN_POINT ( 'NONE',  ( 0.000000000000000000, 4.999999999999999112, 1.000000000000000000 ) ) ;
#18218=DIRECTION ( 'NONE',  ( -0.000000000000000000, -0.000000000000000000, -1.000000000000000000 ) ) ;
#18220=FACE_OUTER_BOUND ( 'NONE', #11281, .T. ) ;
#18221=VECTOR ( 'NONE', #15838, 1000.000000000000000 ) ;
#18223=LINE ( 'NONE', #10167, #7770 ) ;
#18224=LINE ( 'NONE', #6922, #7734 ) ;
#18236=PRODUCT_DEFINITION_CONTEXT ( 'detailed design', #19780, 'design' ) ;
#18237=ORIENTED_EDGE ( 'NONE', *, *, #6489, .F. ) ;
#18238=DIRECTION ( 'NONE',  ( -0.000000000000000000, -0.000000000000000000, -1.000000000000000000 ) ) ;
#18243=CARTESIAN_POINT ( 'NONE',  ( 6.183390479346035917, 0.000000000000000000, 1.000000000000000000 ) ) ;
#18245=DIRECTION ( 'NONE',  ( 0.000000000000000000, -1.000000000000000000, 0.000000000000000000 ) ) ;
#18252=AXIS2_PLACEMENT_3D ( 'NONE', #6323, #12801, #12696 ) ;
#18263=ORIENTED_EDGE ( 'NONE', *, *, #18576, .F. ) ;
#18268=CARTESIAN_POINT ( 'NONE',  ( 11.49178095869207006, 9.000000000000001776, 0.000000000000000000 ) ) ;
#18270=LINE ( 'NONE', #10113, #19661 ) ;
#18273=LINE ( 'NONE', #8758, #5963 ) ;
#18278=VERTEX_POINT ( 'NONE', #10627 ) ;
#18281=VERTEX_POINT ( 'NONE', #4146 ) ;
#18282=VECTOR ( 'NONE', #2730, 1000.000000000000000 ) ;
#18283=EDGE_CURVE ( 'NONE', #487, #16176, #2681, .T. ) ;
#18285=LINE ( 'NONE', #713, #11335 ) ;
#18287=ORIENTED_EDGE ( 'NONE', *, *, #2847, .T. ) ;
#18290=CARTESIAN_POINT ( 'NONE',  ( -7.869520639128047002, 4.999999999999999112, 0.000000000000000000 ) ) ;
#18312=AXIS2_PLACEMENT_3D ( 'NONE', #4463, #18485, #1221 ) ;
#18315=ADVANCED_FACE ( 'NONE', ( #10848 ), #10740, .T. ) ;
#18323=CARTESIAN_POINT ( 'NONE',  ( 1.811130159782011528, 0.000000000000000000, 1.000000000000000000 ) ) ;
#18326=FACE_OUTER_BOUND ( 'NONE', #17035, .T. ) ;
#18335=EDGE_LOOP ( 'NONE', ( #7434, #1641, #2822, #13977 ) ) ;
#18343=DIRECTION ( 'NONE',  ( -0.000000000000000000, 0.000000000000000000, 1.000000000000000000 ) ) ;
#18344=VECTOR ( 'NONE', #18521, 1000.000000000000000 ) ;
#18347=EDGE_CURVE ( 'NONE', #3417, #13354, #18584, .T. ) ;
#18350=DIRECTION ( 'NONE',  ( 1.000000000000000000, 0.000000000000000000, 0.000000000000000000 ) ) ;
#18352=CARTESIAN_POINT ( 'NONE',  ( 27.50000000000000355, 3.000000000000000888, 0.000000000000000000 ) ) ;
#18364=ORIENTED_EDGE ( 'NONE', *, *, #14828, .F. ) ;
#18371=ADVANCED_FACE ( 'NONE', ( #20478 ), #8954, .F. ) ;
#18375=CARTESIAN_POINT ( 'NONE',  ( 23.60856191738414012, 4.999999999999999112, 1.000000000000000000 ) ) ;
#18382=VECTOR ( 'NONE', #63, 1000.000000000000000 ) ;
#18385=DIRECTION ( 'NONE',  ( -0.000000000000000000, -0.000000000000000000, -1.000000000000000000 ) ) ;
#18397=ORIENTED_EDGE ( 'NONE', *, *, #14379, .T. ) ;
#18406=PLANE ( 'NONE',  #8011 ) ;
#18410=AXIS2_PLACEMENT_3D ( 'NONE', #13839, #20242, #14046 ) ;
#18414=CARTESIAN_POINT ( 'NONE',  ( 17.80017143803810242, 9.000000000000001776, 1.000000000000000000 ) ) ;
#18418=VERTEX_POINT ( 'NONE', #9067 ) ;
#18422=EDGE_LOOP ( 'NONE', ( #12418, #9505, #2524, #14700, #10920, #11660, #12446, #14223 ) ) ;
#18423=DIRECTION ( 'NONE',  ( 0.000000000000000000, -1.000000000000000000, 0.000000000000000000 ) ) ;
#18426=VECTOR ( 'NONE', #13194, 1000.000000000000000 ) ;
#18430=EDGE_CURVE ( 'NONE', #3612, #4521, #15439, .T. ) ;
#18431=LINE ( 'NONE', #18533, #11725 ) ;
#18433=CARTESIAN_POINT ( 'NONE',  ( 0.000000000000000000, 9.000000000000001776, 1.000000000000000000 ) ) ;
#18438=ADVANCED_FACE ( 'NONE', ( #8005 ), #6645, .F. ) ;
#18439=AXIS2_PLACEMENT_3D ( 'NONE', #10237, #16603, #2283 ) ;
#18442=ORIENTED_EDGE ( 'NONE', *, *, #2707, .F. ) ;
#18446=PLANE ( 'NONE',  #19706 ) ;
#18448=ORIENTED_EDGE ( 'NONE', *, *, #5819, .F. ) ;
#18449=DIRECTION ( 'NONE',  ( 0.000000000000000000, 1.000000000000000000, 0.000000000000000000 ) ) ;
#18464=DIRECTION ( 'NONE',  ( -0.000000000000000000, -0.000000000000000000, -1.000000000000000000 ) ) ;
#18467=ORIENTED_EDGE ( 'NONE', *, *, #20226, .F. ) ;
#18471=ORIENTED_EDGE ( 'NONE', *, *, #4749, .F. ) ;
#18473=DIRECTION ( 'NONE',  ( 0.000000000000000000, -1.000000000000000000, 0.000000000000000000 ) ) ;
#18478=DIRECTION ( 'NONE',  ( 0.000000000000000000, -1.000000000000000000, 0.000000000000000000 ) ) ;
#18480=ADVANCED_FACE ( 'NONE', ( #12908 ), #11049, .T. ) ;
#18481=DIRECTION ( 'NONE',  ( 1.000000000000000000, 0.000000000000000000, 0.000000000000000000 ) ) ;
#18485=DIRECTION ( 'NONE',  ( 0.000000000000000000, 1.000000000000000000, 0.000000000000000000 ) ) ;
#18487=FACE_OUTER_BOUND ( 'NONE', #17976, .T. ) ;
#18492=ORIENTED_EDGE ( 'NONE', *, *, #8949, .T. ) ;
#18495=ORIENTED_EDGE ( 'NONE', *, *, #12776, .T. ) ;
#18496=AXIS2_PLACEMENT_3D ( 'NONE', #10673, #843, #17045 ) ;
#18497=EDGE_CURVE ( 'NONE', #16676, #5259, #8314, .T. ) ;
#18498=DIRECTION ( 'NONE',  ( -0.000000000000000000, 0.000000000000000000, -1.000000000000000000 ) ) ;
#18499=DIRECTION ( 'NONE',  ( 0.000000000000000000, 1.000000000000000000, 0.000000000000000000 ) ) ;
#18504=DIRECTION ( 'NONE',  ( 0.000000000000000000, -0.000000000000000000, 1.000000000000000000 ) ) ;
#18510=DIRECTION ( 'NONE',  ( 1.000000000000000000, 0.000000000000000000, 0.000000000000000000 ) ) ;
#18519=EDGE_CURVE ( 'NONE', #7330, #9049, #61, .T. ) ;
#18521=DIRECTION ( 'NONE',  ( -0.000000000000000000, -0.000000000000000000, -1.000000000000000000 ) ) ;
#18526=EDGE_LOOP ( 'NONE', ( #9710, #13924, #19946, #12465 ) ) ;
#18533=CARTESIAN_POINT ( 'NONE',  ( 25.04469207716615031, 4.999999999999999112, 1.000000000000000000 ) ) ;
#18539=AXIS2_PLACEMENT_3D ( 'NONE', #1673, #16307, #9515 ) ;
#18545=ORIENTED_EDGE ( 'NONE', *, *, #17724, .T. ) ;
#18549=CIRCLE ( 'NONE', #7254, 0.4999999999999987232 ) ;
#18555=CARTESIAN_POINT ( 'NONE',  ( 0.000000000000000000, 9.000000000000001776, 1.000000000000000000 ) ) ;
#18561=CARTESIAN_POINT ( 'NONE',  ( -13.17791111847408025, 0.000000000000000000, 1.000000000000000000 ) ) ;
#18567=ORIENTED_EDGE ( 'NONE', *, *, #16928, .F. ) ;
#18569=ORIENTED_EDGE ( 'NONE', *, *, #1949, .T. ) ;
#18574=CARTESIAN_POINT ( 'NONE',  ( -13.67767524182159100, -0.4755849646238735073, 1.001433380786713068 ) ) ;
#18575=ADVANCED_FACE ( 'NONE', ( #9475 ), #14581, .T. ) ;
#18576=EDGE_CURVE ( 'NONE', #1583, #18591, #9782, .T. ) ;
#18577=EDGE_LOOP ( 'NONE', ( #5709, #16184, #13750, #11206 ) ) ;
#18578=DIRECTION ( 'NONE',  ( -1.734723475976807094E-15, 1.000000000000000000, 0.000000000000000000 ) ) ;
#18579=CARTESIAN_POINT ( 'NONE',  ( 23.60856191738414012, 0.000000000000000000, 1.000000000000000000 ) ) ;
#18584=LINE ( 'NONE', #10529, #270 ) ;
#18586=DIRECTION ( 'NONE',  ( 1.000000000000000000, 0.000000000000000000, -0.000000000000000000 ) ) ;
#18591=VERTEX_POINT ( 'NONE', #16169 ) ;
#18594=EDGE_LOOP ( 'NONE', ( #18982, #4540, #4890, #686 ) ) ;
#18595=DIRECTION ( 'NONE',  ( -0.000000000000000000, -0.000000000000000000, -1.000000000000000000 ) ) ;
#18597=FACE_OUTER_BOUND ( 'NONE', #13162, .T. ) ;
#18600=ORIENTED_EDGE ( 'NONE', *, *, #7773, .T. ) ;
#18606=CARTESIAN_POINT ( 'NONE',  ( 3.999999999999999112, -2.500000000000047518, 7.000000000000000000 ) ) ;
#18613=B_SPLINE_CURVE_WITH_KNOTS ( 'NONE', 3,
 ( #2781, #15527, #18574, #1417, #14161, #20568, #6220, #5912, #15036, #2670 ),
 .UNSPECIFIED., .F., .F.,
 ( 4, 2, 2, 2, 4 ),
 ( 0.000000000000000000, 0.0002648908096818753050, 0.0005297816193637506100, 0.0007946724290456259150, 0.001059563238727501437 ),
 .UNSPECIFIED. ) ;
#18621=ORIENTED_EDGE ( 'NONE', *, *, #20498, .T. ) ;
#18622=EDGE_CURVE ( 'NONE', #12851, #17198, #14267, .T. ) ;
#18623=ORIENTED_EDGE ( 'NONE', *, *, #13710, .T. ) ;
#18625=LINE ( 'NONE', #7634, #11471 ) ;
#18629=VERTEX_POINT ( 'NONE', #12708 ) ;
#18632=LINE ( 'NONE', #2835, #6149 ) ;
#18634=EDGE_CURVE ( 'NONE', #5490, #18833, #4763, .T. ) ;
#18637=DIRECTION ( 'NONE',  ( 1.000000000000000000, 0.000000000000000000, 0.000000000000000000 ) ) ;
#18646=ORIENTED_EDGE ( 'NONE', *, *, #20385, .F. ) ;
#18654=EDGE_CURVE ( 'NONE', #4981, #68, #8427, .T. ) ;
#18656=FACE_OUTER_BOUND ( 'NONE', #18836, .T. ) ;
#18657=DIRECTION ( 'NONE',  ( 1.000000000000000000, 0.000000000000000000, 0.000000000000000000 ) ) ;
#18662=ORIENTED_EDGE ( 'NONE', *, *, #11946, .T. ) ;
#18667=ORIENTED_EDGE ( 'NONE', *, *, #14598, .T. ) ;
#18669=DIRECTION ( 'NONE',  ( -0.000000000000000000, 0.000000000000000000, -1.000000000000000000 ) ) ;
#18670=VECTOR ( 'NONE', #3731, 1000.000000000000000 ) ;
#18672=AXIS2_PLACEMENT_3D ( 'NONE', #4265, #5744, #12115 ) ;
#18675=VECTOR ( 'NONE', #2339, 1000.000000000000000 ) ;
#18682=LINE ( 'NONE', #13446, #7675 ) ;
#18683=DIRECTION ( 'NONE',  ( 0.000000000000000000, 1.000000000000000000, -0.000000000000000000 ) ) ;
#18684=VECTOR ( 'NONE', #6327, 1000.000000000000000 ) ;
#18692=DIRECTION ( 'NONE',  ( 0.000000000000000000, 0.000000000000000000, 1.000000000000000000 ) ) ;
#18698=ADVANCED_FACE ( 'NONE', ( #8733 ), #6949, .T. ) ;
#18704=ORIENTED_EDGE ( 'NONE', *, *, #9541, .F. ) ;
#18708=ORIENTED_EDGE ( 'NONE', *, *, #553, .T. ) ;
#18711=CIRCLE ( 'NONE', #18047, 0.5000000000000000000 ) ;
#18714=LINE ( 'NONE', #18820, #8966 ) ;
#18725=AXIS2_PLACEMENT_3D ( 'NONE', #3469, #5142, #9947 ) ;
#18727=DIRECTION ( 'NONE',  ( 1.000000000000000000, 0.000000000000000000, 0.000000000000000000 ) ) ;
#18728=EDGE_LOOP ( 'NONE', ( #15774, #13414, #4030, #17126 ) ) ;
#18731=CARTESIAN_POINT ( 'NONE',  ( 0.000000000000000000, 4.999999999999999112, 0.000000000000000000 ) ) ;
#18732=( LENGTH_UNIT ( ) NAMED_UNIT ( * ) SI_UNIT ( .MILLI., .METRE. ) );
#18734=LINE ( 'NONE', #7541, #19493 ) ;
#18737=PLANE ( 'NONE',  #18957 ) ;
#18742=ADVANCED_FACE ( 'NONE', ( #4017 ), #13123, .F. ) ;
#18743=EDGE_CURVE ( 'NONE', #13273, #9411, #9980, .T. ) ;
#18744=LINE ( 'NONE', #15584, #2041 ) ;
#18754=VECTOR ( 'NONE', #11103, 1000.000000000000000 ) ;
#18756=ORIENTED_EDGE ( 'NONE', *, *, #664, .T. ) ;
#18759=ORIENTED_EDGE ( 'NONE', *, *, #14329, .F. ) ;
#18760=FACE_OUTER_BOUND ( 'NONE', #10753, .T. ) ;
#18767=CARTESIAN_POINT ( 'NONE',  ( 11.49178095869207006, 9.000000000000001776, 1.000000000000000000 ) ) ;
#18775=DIRECTION ( 'NONE',  ( -0.000000000000000000, -0.000000000000000000, -1.000000000000000000 ) ) ;
#18780=PLANE ( 'NONE',  #10057 ) ;
#18791=DIRECTION ( 'NONE',  ( -0.000000000000000000, -0.000000000000000000, -1.000000000000000000 ) ) ;
#18792=CARTESIAN_POINT ( 'NONE',  ( -11.74178095869206828, 9.000000000000001776, 1.000000000000000000 ) ) ;
#18796=VECTOR ( 'NONE', #6015, 1000.000000000000000 ) ;
#18797=DIRECTION ( 'NONE',  ( -0.000000000000000000, -0.000000000000000000, -1.000000000000000000 ) ) ;
#18803=VECTOR ( 'NONE', #18138, 1000.000000000000000 ) ;
#18807=DIRECTION ( 'NONE',  ( -0.000000000000000000, -0.000000000000000000, -1.000000000000000000 ) ) ;
#18810=VERTEX_POINT ( 'NONE', #778 ) ;
#18814=DIRECTION ( 'NONE',  ( 0.7071067811865474617, -0.000000000000000000, 0.7071067811865474617 ) ) ;
#18817=ADVANCED_FACE ( 'NONE', ( #3601 ), #673, .T. ) ;
#18820=CARTESIAN_POINT ( 'NONE',  ( 0.000000000000000000, 9.000000000000001776, 0.000000000000000000 ) ) ;
#18824=( NAMED_UNIT ( * ) SI_UNIT ( $, .STERADIAN. ) SOLID_ANGLE_UNIT ( ) );
#18828=DIRECTION ( 'NONE',  ( 0.000000000000000000, -0.000000000000000000, 1.000000000000000000 ) ) ;
#18832=EDGE_LOOP ( 'NONE', ( #11863, #8327, #12086, #13778 ) ) ;
#18833=VERTEX_POINT ( 'NONE', #18352 ) ;
#18835=CARTESIAN_POINT ( 'NONE',  ( 4.247260319564023945, 9.000000000000001776, 1.000000000000000000 ) ) ;
#18836=EDGE_LOOP ( 'NONE', ( #16274, #17795, #20240, #685 ) ) ;
#18838=PLANE ( 'NONE',  #2112 ) ;
#18841=CARTESIAN_POINT ( 'NONE',  ( 0.000000000000000000, 4.999999999999999112, 1.000000000000000000 ) ) ;
#18847=FACE_OUTER_BOUND ( 'NONE', #4187, .T. ) ;
#18856=ORIENTED_EDGE ( 'NONE', *, *, #14523, .T. ) ;
#18862=LINE ( 'NONE', #10908, #14112 ) ;
#18870=LINE ( 'NONE', #17704, #12396 ) ;
#18884=LINE ( 'NONE', #1693, #13107 ) ;
#18895=DIRECTION ( 'NONE',  ( 1.000000000000000000, 0.000000000000000000, 0.000000000000000000 ) ) ;
#18899=EDGE_CURVE ( 'NONE', #3823, #15395, #980, .T. ) ;
#18902=LINE ( 'NONE', #17212, #19709 ) ;
#18911=EDGE_LOOP ( 'NONE', ( #11493, #3616, #7674, #7931 ) ) ;
#18912=CARTESIAN_POINT ( 'NONE',  ( 0.000000000000000000, 0.000000000000000000, 1.000000000000000000 ) ) ;
#18920=DIRECTION ( 'NONE',  ( 0.000000000000000000, 1.000000000000000000, -0.000000000000000000 ) ) ;
#18922=DIRECTION ( 'NONE',  ( 0.000000000000000000, 1.000000000000000000, 0.000000000000000000 ) ) ;
#18926=ADVANCED_FACE ( 'NONE', ( #4435 ), #12375, .T. ) ;
#18932=DIRECTION ( 'NONE',  ( 0.000000000000000000, 1.000000000000000000, -0.000000000000000000 ) ) ;
#18936=( NAMED_UNIT ( * ) SI_UNIT ( $, .STERADIAN. ) SOLID_ANGLE_UNIT ( ) );
#18939=ORIENTED_EDGE ( 'NONE', *, *, #13338, .T. ) ;
#18950=DIRECTION ( 'NONE',  ( -0.000000000000000000, 0.000000000000000000, 1.000000000000000000 ) ) ;
#18954=ORIENTED_EDGE ( 'NONE', *, *, #12553, .F. ) ;
#18955=EDGE_CURVE ( 'NONE', #4851, #7250, #15609, .T. ) ;
#18957=AXIS2_PLACEMENT_3D ( 'NONE', #4404, #10383, #6386 ) ;
#18971=CARTESIAN_POINT ( 'NONE',  ( 17.30017143803810242, 0.000000000000000000, 1.000000000000000000 ) ) ;
#18973=ADVANCED_FACE ( 'NONE', ( #3781 ), #5553, .T. ) ;
#18979=VECTOR ( 'NONE', #17967, 1000.000000000000000 ) ;
#18982=ORIENTED_EDGE ( 'NONE', *, *, #19098, .F. ) ;
#18984=CARTESIAN_POINT ( 'NONE',  ( 14.00000000000000000, 7.806255641895631925E-15, 1.000000000000000000 ) ) ;
#18985=LINE ( 'NONE', #11033, #10005 ) ;
#18988=DIRECTION ( 'NONE',  ( -0.000000000000000000, -1.000000000000000000, -0.000000000000000000 ) ) ;
#18993=CARTESIAN_POINT ( 'NONE',  ( -5.999999999999999112, -7.500000000000047073, 9.999999999999998224 ) ) ;
#18999=EDGE_CURVE ( 'NONE', #2052, #5735, #15172, .T. ) ;
#19002=EDGE_CURVE ( 'NONE', #16377, #9583, #10159, .T. ) ;
#19010=ADVANCED_FACE ( 'NONE', ( #14957 ), #2413, .T. ) ;
#19014=EDGE_LOOP ( 'NONE', ( #5514, #1896, #5621, #15906, #6866, #6881, #2806, #4978, #17449, #17495, #16570, #3033, #10389, #18623, #9199, #15597, #8026, #18027, #9690, #4029, #18708, #11559, #8235, #15700, #16291, #12015, #11790, #14571, #7532, #13871, #16875, #9940, #5832, #15312, #20145, #1208, #10517, #12387, #16501, #19373, #7990, #19737, #13110, #19222, #8667, #10874, #17460, #5028, #14953, #15658, #5983, #892, #15755, #5161, #744, #20194, #16548, #7814, #3002, #13836, #20400, #557, #17238, #15449, #11763, #6221, #10469, #3112, #11740, #17748, #19869, #9486, #9002, #652, #8887, #16609, #20494, #17609, #3137, #16615, #12130, #13206, #10840, #19017, #18662, #3210, #9580, #7533, #1717, #3998, #14363, #8872, #1934, #5915, #6536, #5986, #5525, #6539, #15290, #7635, #8274, #15446, #19833, #325, #17820, #10133, #9178, #781, #11714, #8125, #10782, #6042, #156, #358, #17148, #15146, #8153, #8634, #19149, #14298 ) ) ;
#19017=ORIENTED_EDGE ( 'NONE', *, *, #8465, .T. ) ;
#19019=EDGE_CURVE ( 'NONE', #19533, #5029, #13187, .T. ) ;
#19021=VERTEX_POINT ( 'NONE', #2106 ) ;
#19030=CARTESIAN_POINT ( 'NONE',  ( -9.805650798910056309, 4.999999999999999112, 0.000000000000000000 ) ) ;
#19034=VECTOR ( 'NONE', #14816, 1000.000000000000000 ) ;
#19038=LINE ( 'NONE', #4695, #6626 ) ;
#19043=DIRECTION ( 'NONE',  ( 0.000000000000000000, 1.000000000000000000, -0.000000000000000000 ) ) ;
#19045=EDGE_CURVE ( 'NONE', #8332, #3444, #19682, .T. ) ;
#19047=ORIENTED_EDGE ( 'NONE', *, *, #10755, .T. ) ;
#19050=DIRECTION ( 'NONE',  ( 0.000000000000000000, 0.000000000000000000, 1.000000000000000000 ) ) ;
#19052=( GEOMETRIC_REPRESENTATION_CONTEXT ( 3 ) GLOBAL_UNCERTAINTY_ASSIGNED_CONTEXT ( ( #1081 ) ) GLOBAL_UNIT_ASSIGNED_CONTEXT ( ( #17353, #15681, #18936 ) ) REPRESENTATION_CONTEXT ( 'NONE', 'WORKASPACE' ) );
#19053=CARTESIAN_POINT ( 'NONE',  ( 25.54469207716615031, 9.000000000000001776, 1.000000000000000000 ) ) ;
#19066=ORIENTED_EDGE ( 'NONE', *, *, #3665, .F. ) ;
#19067=DIRECTION ( 'NONE',  ( -1.734723475976807094E-15, 1.000000000000000000, 0.000000000000000000 ) ) ;
#19082=ORIENTED_EDGE ( 'NONE', *, *, #13066, .F. ) ;
#19089=VERTEX_POINT ( 'NONE', #8694 ) ;
#19093=CARTESIAN_POINT ( 'NONE',  ( -3.497260319564023057, 9.000000000000001776, 1.000000000000000000 ) ) ;
#19095=VERTEX_POINT ( 'NONE', #2303 ) ;
#19098=EDGE_CURVE ( 'NONE', #17042, #17247, #13282, .T. ) ;
#19100=VECTOR ( 'NONE', #521, 1000.000000000000000 ) ;
#19101=CARTESIAN_POINT ( 'NONE',  ( 15.36404127825609400, 4.999999999999999112, 1.000000000000000000 ) ) ;
#19103=VECTOR ( 'NONE', #6727, 1000.000000000000000 ) ;
#19104=CARTESIAN_POINT ( 'NONE',  ( 15.36404127825609400, 4.999999999999999112, 1.000000000000000000 ) ) ;
#19110=CARTESIAN_POINT ( 'NONE',  ( -15.11404127825609223, 0.000000000000000000, 0.000000000000000000 ) ) ;
#19115=EDGE_CURVE ( 'NONE', #13902, #7075, #4090, .T. ) ;
#19120=CARTESIAN_POINT ( 'NONE',  ( 19.73630159782011617, 4.999999999999999112, 1.000000000000000000 ) ) ;
#19121=ORIENTED_EDGE ( 'NONE', *, *, #13827, .T. ) ;
#19123=CARTESIAN_POINT ( 'NONE',  ( 3.999999999999999112, -7.500000000000047073, 2.000000000000000000 ) ) ;
#19125=CARTESIAN_POINT ( 'NONE',  ( -5.933390479346035029, 0.000000000000000000, 0.000000000000000000 ) ) ;
#19129=VERTEX_POINT ( 'NONE', #7230 ) ;
#19131=DIRECTION ( 'NONE',  ( 1.000000000000000000, 0.000000000000000000, 0.000000000000000000 ) ) ;
#19135=AXIS2_PLACEMENT_3D ( 'NONE', #14498, #6770, #3213 ) ;
#19139=EDGE_CURVE ( 'NONE', #6961, #7639, #8804, .T. ) ;
#19143=DIRECTION ( 'NONE',  ( 0.000000000000000000, 1.000000000000000000, -0.000000000000000000 ) ) ;
#19146=LINE ( 'NONE', #14518, #302 ) ;
#19147=VERTEX_POINT ( 'NONE', #16530 ) ;
#19149=ORIENTED_EDGE ( 'NONE', *, *, #7123, .T. ) ;
#19160=DIRECTION ( 'NONE',  ( 1.000000000000000000, 0.000000000000000000, -0.000000000000000000 ) ) ;
#19166=CARTESIAN_POINT ( 'NONE',  ( 17.30017143803810242, 9.000000000000001776, 0.000000000000000000 ) ) ;
#19171=VERTEX_POINT ( 'NONE', #15580 ) ;
#19176=CARTESIAN_POINT ( 'NONE',  ( 11.99178095869207006, 4.999999999999999112, 1.000000000000000000 ) ) ;
#19179=LINE ( 'NONE', #4832, #7260 ) ;
#19181=PLANE ( 'NONE',  #8024 ) ;
#19188=ORIENTED_EDGE ( 'NONE', *, *, #13469, .F. ) ;
#19197=PLANE ( 'NONE',  #2659 ) ;
#19204=DIRECTION ( 'NONE',  ( -0.000000000000000000, -0.000000000000000000, -1.000000000000000000 ) ) ;
#19206=PLANE ( 'NONE',  #1850 ) ;
#19210=DIRECTION ( 'NONE',  ( 0.000000000000000000, 0.000000000000000000, 1.000000000000000000 ) ) ;
#19222=ORIENTED_EDGE ( 'NONE', *, *, #16512, .T. ) ;
#19223=CARTESIAN_POINT ( 'NONE',  ( 0.000000000000000000, 4.999999999999999112, 0.000000000000000000 ) ) ;
#19226=EDGE_CURVE ( 'NONE', #13134, #3417, #19672, .T. ) ;
#19227=EDGE_CURVE ( 'NONE', #2846, #7153, #13487, .T. ) ;
#19241=ORIENTED_EDGE ( 'NONE', *, *, #11128, .T. ) ;
#19243=CARTESIAN_POINT ( 'NONE',  ( -27.50000000000000711, 4.999999999999999112, 1.000000000000000000 ) ) ;
#19251=CARTESIAN_POINT ( 'NONE',  ( 13.42791111847407848, 9.000000000000001776, 1.000000000000000000 ) ) ;
#19259=DIRECTION ( 'NONE',  ( 0.000000000000000000, -0.000000000000000000, 1.000000000000000000 ) ) ;
#19271=EDGE_LOOP ( 'NONE', ( #10545, #3039, #14228, #11867 ) ) ;
#19277=LINE ( 'NONE', #6194, #16787 ) ;
#19281=DIRECTION ( 'NONE',  ( -0.7071067811865474617, -0.000000000000000000, 0.7071067811865474617 ) ) ;
#19287=DIRECTION ( 'NONE',  ( -0.000000000000000000, -0.000000000000000000, -1.000000000000000000 ) ) ;
#19290=ORIENTED_EDGE ( 'NONE', *, *, #6440, .T. ) ;
#19293=CARTESIAN_POINT ( 'NONE',  ( -24.79469207716615031, 4.999999999999999112, 0.000000000000000000 ) ) ;
#19299=LINE ( 'NONE', #8204, #2327 ) ;
#19300=ORIENTED_EDGE ( 'NONE', *, *, #5565, .F. ) ;
#19303=EDGE_CURVE ( 'NONE', #7476, #19147, #4079, .T. ) ;
#19306=CARTESIAN_POINT ( 'NONE',  ( -3.997260319564023501, 0.000000000000000000, 1.000000000000000000 ) ) ;
#19308=DIRECTION ( 'NONE',  ( -0.000000000000000000, 0.000000000000000000, -1.000000000000000000 ) ) ;
#19311=LINE ( 'NONE', #6544, #9697 ) ;
#19312=DIRECTION ( 'NONE',  ( 0.000000000000000000, 0.000000000000000000, 1.000000000000000000 ) ) ;
#19330=EDGE_CURVE ( 'NONE', #11328, #15500, #8578, .T. ) ;
#19331=LINE ( 'NONE', #4989, #18670 ) ;
#19332=CARTESIAN_POINT ( 'NONE',  ( -13.17791111847408025, 4.999999999999999112, 1.000000000000000000 ) ) ;
#19335=CARTESIAN_POINT ( 'NONE',  ( 0.000000000000000000, 9.000000000000001776, 0.000000000000000000 ) ) ;
#19337=ADVANCED_FACE ( 'NONE', ( #19786 ), #8894, .T. ) ;
#19339=DIRECTION ( 'NONE',  ( 0.000000000000000000, 1.000000000000000000, -0.000000000000000000 ) ) ;
#19347=CARTESIAN_POINT ( 'NONE',  ( -17.55017143803810242, 0.000000000000000000, 1.000000000000000000 ) ) ;
#19350=ORIENTED_EDGE ( 'NONE', *, *, #6908, .F. ) ;
#19366=AXIS2_PLACEMENT_3D ( 'NONE', #8770, #16593, #816 ) ;
#19367=DIRECTION ( 'NONE',  ( 1.000000000000000000, 1.192622389734054877E-16, -0.000000000000000000 ) ) ;
#19373=ORIENTED_EDGE ( 'NONE', *, *, #7251, .T. ) ;
#19379=DIRECTION ( 'NONE',  ( 0.000000000000000000, 1.000000000000000000, -0.000000000000000000 ) ) ;
#19384=ADVANCED_FACE ( 'NONE', ( #15163 ), #13686, .T. ) ;
#19393=DIRECTION ( 'NONE',  ( 0.000000000000000000, 1.000000000000000000, -0.000000000000000000 ) ) ;
#19394=VECTOR ( 'NONE', #1805, 1000.000000000000000 ) ;
#19395=EDGE_LOOP ( 'NONE', ( #355, #13585, #20486, #14179 ) ) ;
#19405=ORIENTED_EDGE ( 'NONE', *, *, #927, .F. ) ;
#19412=LINE ( 'NONE', #19306, #18684 ) ;
#19414=CARTESIAN_POINT ( 'NONE',  ( 4.999999999999998224, -2.500000000000047518, 9.999999999999998224 ) ) ;
#19423=VERTEX_POINT ( 'NONE', #14201 ) ;
#19430=DIRECTION ( 'NONE',  ( -0.000000000000000000, -0.000000000000000000, -1.000000000000000000 ) ) ;
#19431=ORIENTED_EDGE ( 'NONE', *, *, #16803, .F. ) ;
#19436=VECTOR ( 'NONE', #15895, 1000.000000000000000 ) ;
#19438=ORIENTED_EDGE ( 'NONE', *, *, #19227, .T. ) ;
#19440=CARTESIAN_POINT ( 'NONE',  ( 0.000000000000000000, 4.999999999999999112, 1.000000000000000000 ) ) ;
#19442=CARTESIAN_POINT ( 'NONE',  ( 0.000000000000000000, 9.000000000000001776, 1.000000000000000000 ) ) ;
#19453=ADVANCED_FACE ( 'NONE', ( #1154 ), #15571, .T. ) ;
#19454=DIRECTION ( 'NONE',  ( 0.000000000000000000, 0.000000000000000000, -1.000000000000000000 ) ) ;
#19455=LINE ( 'NONE', #11383, #3316 ) ;
#19456=VECTOR ( 'NONE', #2336, 1000.000000000000000 ) ;
#19463=VECTOR ( 'NONE', #17409, 1000.000000000000000 ) ;
#19476=VECTOR ( 'NONE', #4110, 1000.000000000000000 ) ;
#19477=ADVANCED_FACE ( 'NONE', ( #1361 ), #6167, .T. ) ;
#19481=EDGE_LOOP ( 'NONE', ( #7817, #8962, #17119, #6585 ) ) ;
#19483=DIRECTION ( 'NONE',  ( -0.000000000000000000, -0.000000000000000000, -1.000000000000000000 ) ) ;
#19488=EDGE_CURVE ( 'NONE', #17662, #14732, #2980, .T. ) ;
#19489=FACE_OUTER_BOUND ( 'NONE', #168, .T. ) ;
#19491=CARTESIAN_POINT ( 'NONE',  ( 0.000000000000000000, 4.999999999999999112, 1.000000000000000000 ) ) ;
#19492=EDGE_CURVE ( 'NONE', #10573, #20689, #6261, .T. ) ;
#19493=VECTOR ( 'NONE', #2411, 1000.000000000000000 ) ;
#19502=EDGE_CURVE ( 'NONE', #9491, #12176, #12634, .T. ) ;
#19506=ORIENTED_EDGE ( 'NONE', *, *, #18955, .T. ) ;
#19517=DIRECTION ( 'NONE',  ( 0.000000000000000000, 1.000000000000000000, 0.000000000000000000 ) ) ;
#19518=LINE ( 'NONE', #17930, #11737 ) ;
#19519=DIRECTION ( 'NONE',  ( 0.1736481776669295540, 0.9848077530122082424, 0.000000000000000000 ) ) ;
#19520=CARTESIAN_POINT ( 'NONE',  ( 0.000000000000000000, 9.000000000000001776, 0.000000000000000000 ) ) ;
#19526=EDGE_CURVE ( 'NONE', #734, #458, #20297, .T. ) ;
#19531=DIRECTION ( 'NONE',  ( 0.000000000000000000, 0.000000000000000000, -1.000000000000000000 ) ) ;
#19533=VERTEX_POINT ( 'NONE', #12229 ) ;
#19534=PLANE ( 'NONE',  #3714 ) ;
#19538=DIRECTION ( 'NONE',  ( -0.000000000000000000, -0.000000000000000000, -1.000000000000000000 ) ) ;
#19542=DIRECTION ( 'NONE',  ( 1.000000000000000000, 0.000000000000000000, 0.000000000000000000 ) ) ;
#19543=DIRECTION ( 'NONE',  ( 1.000000000000000000, 0.000000000000000000, 0.000000000000000000 ) ) ;
#19546=CARTESIAN_POINT ( 'NONE',  ( -20.00000000000000000, -0.5000000000000004441, 1.000000000000000000 ) ) ;
#19548=VERTEX_POINT ( 'NONE', #10777 ) ;
#19552=ORIENTED_EDGE ( 'NONE', *, *, #3626, .F. ) ;
#19553=DIRECTION ( 'NONE',  ( -0.000000000000000000, -1.000000000000000000, -0.000000000000000000 ) ) ;
#19554=CARTESIAN_POINT ( 'NONE',  ( 8.119520639128047890, 4.999999999999999112, 1.000000000000000000 ) ) ;
#19555=ORIENTED_EDGE ( 'NONE', *, *, #6908, .T. ) ;
#19556=SHAPE_DEFINITION_REPRESENTATION ( #1328, #537 ) ;
#19557=ORIENTED_EDGE ( 'NONE', *, *, #12309, .F. ) ;
#19559=AXIS2_PLACEMENT_3D ( 'NONE', #19491, #10935, #9467 ) ;
#19579=DIRECTION ( 'NONE',  ( -0.000000000000000000, -0.000000000000000000, -1.000000000000000000 ) ) ;
#19583=CARTESIAN_POINT ( 'NONE',  ( 0.000000000000000000, 4.999999999999999112, 0.000000000000000000 ) ) ;
#19587=VECTOR ( 'NONE', #6676, 1000.000000000000000 ) ;
#19600=VERTEX_POINT ( 'NONE', #6579 ) ;
#19604=ORIENTED_EDGE ( 'NONE', *, *, #4886, .F. ) ;
#19607=CARTESIAN_POINT ( 'NONE',  ( 24.50000000000000000, 3.000000000000000888, 1.000000000000000000 ) ) ;
#19609=EDGE_CURVE ( 'NONE', #11516, #4449, #19146, .T. ) ;
#19613=LINE ( 'NONE', #2035, #4724 ) ;
#19624=CARTESIAN_POINT ( 'NONE',  ( -9.305650798910056309, 9.000000000000001776, 1.000000000000000000 ) ) ;
#19625=VERTEX_POINT ( 'NONE', #15981 ) ;
#19628=CARTESIAN_POINT ( 'NONE',  ( -22.85856191738413656, 0.000000000000000000, 0.000000000000000000 ) ) ;
#19629=ORIENTED_EDGE ( 'NONE', *, *, #18622, .F. ) ;
#19633=CARTESIAN_POINT ( 'NONE',  ( -15.61404127825609223, 9.000000000000001776, 0.000000000000000000 ) ) ;
#19634=EDGE_CURVE ( 'NONE', #10100, #8356, #6483, .T. ) ;
#19635=EDGE_CURVE ( 'NONE', #15500, #4847, #11491, .T. ) ;
#19640=FACE_OUTER_BOUND ( 'NONE', #16352, .T. ) ;
#19642=LINE ( 'NONE', #8548, #1539 ) ;
#19645=VERTEX_POINT ( 'NONE', #3540 ) ;
#19648=VERTEX_POINT ( 'NONE', #19554 ) ;
#19651=CARTESIAN_POINT ( 'NONE',  ( -17.05017143803810242, 0.000000000000000000, 0.000000000000000000 ) ) ;
#19653=ORIENTED_EDGE ( 'NONE', *, *, #15426, .T. ) ;
#19654=CARTESIAN_POINT ( 'NONE',  ( 1.811130159782011528, 9.000000000000001776, 0.000000000000000000 ) ) ;
#19655=ORIENTED_EDGE ( 'NONE', *, *, #14331, .F. ) ;
#19660=CARTESIAN_POINT ( 'NONE',  ( -2.061130159782011972, 9.000000000000001776, 1.000000000000000000 ) ) ;
#19661=VECTOR ( 'NONE', #19543, 1000.000000000000000 ) ;
#19664=DIRECTION ( 'NONE',  ( -1.000000000000000000, 0.000000000000000000, 0.000000000000000000 ) ) ;
#19670=EDGE_CURVE ( 'NONE', #11975, #7606, #1662, .T. ) ;
#19672=LINE ( 'NONE', #2605, #2643 ) ;
#19675=EDGE_LOOP ( 'NONE', ( #3107, #10152, #4258, #8483 ) ) ;
#19681=DIRECTION ( 'NONE',  ( -0.000000000000000000, 1.000000000000000000, -0.000000000000000000 ) ) ;
#19682=LINE ( 'NONE', #5238, #6638 ) ;
#19686=PLANE ( 'NONE',  #1513 ) ;
#19688=AXIS2_PLACEMENT_3D ( 'NONE', #13584, #19985, #2499 ) ;
#19702=VECTOR ( 'NONE', #5606, 1000.000000000000000 ) ;
#19706=AXIS2_PLACEMENT_3D ( 'NONE', #3898, #5680, #20123 ) ;
#19707=ORIENTED_EDGE ( 'NONE', *, *, #5615, .T. ) ;
#19708=DIRECTION ( 'NONE',  ( 1.000000000000000000, 0.000000000000000000, 0.000000000000000000 ) ) ;
#19709=VECTOR ( 'NONE', #15638, 1000.000000000000000 ) ;
#19712=ADVANCED_FACE ( 'NONE', ( #5002 ), #8156, .T. ) ;
#19716=PLANE ( 'NONE',  #8396 ) ;
#19720=DIRECTION ( 'NONE',  ( -1.013672804646636192E-16, 1.000000000000000000, 0.000000000000000000 ) ) ;
#19723=ORIENTED_EDGE ( 'NONE', *, *, #6571, .T. ) ;
#19728=ORIENTED_EDGE ( 'NONE', *, *, #11418, .F. ) ;
#19730=LINE ( 'NONE', #15311, #5366 ) ;
#19731=VERTEX_POINT ( 'NONE', #12744 ) ;
#19737=ORIENTED_EDGE ( 'NONE', *, *, #14456, .T. ) ;
#19738=EDGE_CURVE ( 'NONE', #610, #20018, #19455, .T. ) ;
#19743=LINE ( 'NONE', #19440, #2977 ) ;
#19744=VECTOR ( 'NONE', #1222, 1000.000000000000000 ) ;
#19749=DIRECTION ( 'NONE',  ( 0.000000000000000000, 1.000000000000000000, -0.000000000000000000 ) ) ;
#19754=ORIENTED_EDGE ( 'NONE', *, *, #11934, .T. ) ;
#19758=VECTOR ( 'NONE', #19287, 1000.000000000000000 ) ;
#19760=ADVANCED_FACE ( 'NONE', ( #16204 ), #6376, .T. ) ;
#19761=FACE_OUTER_BOUND ( 'NONE', #15157, .T. ) ;
#19766=VERTEX_POINT ( 'NONE', #4898 ) ;
#19775=LINE ( 'NONE', #728, #1400 ) ;
#19776=CARTESIAN_POINT ( 'NONE',  ( -5.933390479346035029, 9.000000000000001776, 1.000000000000000000 ) ) ;
#19780=APPLICATION_CONTEXT ( 'automotive_design' ) ;
#19786=FACE_OUTER_BOUND ( 'NONE', #7992, .T. ) ;
#19788=EDGE_CURVE ( 'NONE', #9899, #485, #9714, .T. ) ;
#19789=VERTEX_POINT ( 'NONE', #10333 ) ;
#19794=VECTOR ( 'NONE', #18988, 1000.000000000000000 ) ;
#19796=CARTESIAN_POINT ( 'NONE',  ( -7.369520639128046113, 4.999999999999999112, 1.000000000000000000 ) ) ;
#19797=DIRECTION ( 'NONE',  ( 0.000000000000000000, 1.000000000000000000, 0.000000000000000000 ) ) ;
#19802=VECTOR ( 'NONE', #2557, 1000.000000000000000 ) ;
#19818=ORIENTED_EDGE ( 'NONE', *, *, #18283, .F. ) ;
#19819=VERTEX_POINT ( 'NONE', #5520 ) ;
#19821=VECTOR ( 'NONE', #18238, 1000.000000000000000 ) ;
#19827=DIRECTION ( 'NONE',  ( -0.000000000000000000, -0.000000000000000000, -1.000000000000000000 ) ) ;
#19833=ORIENTED_EDGE ( 'NONE', *, *, #3640, .T. ) ;
#19844=ORIENTED_EDGE ( 'NONE', *, *, #12067, .F. ) ;
#19849=CARTESIAN_POINT ( 'NONE',  ( -21.42243175760212637, 9.000000000000001776, 1.000000000000000000 ) ) ;
#19850=CARTESIAN_POINT ( 'NONE',  ( -9.805650798910056309, 9.000000000000001776, 1.000000000000000000 ) ) ;
#19851=CARTESIAN_POINT ( 'NONE',  ( -17.11324865405191176, -11.00000000000000000, 2.000000000000000000 ) ) ;
#19854=ADVANCED_FACE ( 'NONE', ( #8556 ), #19868, .F. ) ;
#19861=ORIENTED_EDGE ( 'NONE', *, *, #10636, .F. ) ;
#19862=EDGE_CURVE ( 'NONE', #12057, #16179, #18285, .T. ) ;
#19866=ADVANCED_FACE ( 'NONE', ( #16402 ), #15031, .F. ) ;
#19868=PLANE ( 'NONE',  #8665 ) ;
#19869=ORIENTED_EDGE ( 'NONE', *, *, #18347, .T. ) ;
#19870=ORIENTED_EDGE ( 'NONE', *, *, #17797, .F. ) ;
#19871=ORIENTED_EDGE ( 'NONE', *, *, #12470, .F. ) ;
#19875=PLANE ( 'NONE',  #13694 ) ;
#19884=CARTESIAN_POINT ( 'NONE',  ( -11.24178095869206828, 9.000000000000001776, 1.000000000000000000 ) ) ;
#19885=LINE ( 'NONE', #4076, #7077 ) ;
#19893=DIRECTION ( 'NONE',  ( -0.000000000000000000, 0.000000000000000000, -1.000000000000000000 ) ) ;
#19895=DIRECTION ( 'NONE',  ( 0.000000000000000000, 1.000000000000000000, -0.000000000000000000 ) ) ;
#19896=DIRECTION ( 'NONE',  ( 0.000000000000000000, 1.000000000000000000, 0.000000000000000000 ) ) ;
#19897=CARTESIAN_POINT ( 'NONE',  ( 10.05565079891005631, 9.000000000000001776, 1.000000000000000000 ) ) ;
#19899=PLANE ( 'NONE',  #14187 ) ;
#19901=EDGE_CURVE ( 'NONE', #20292, #740, #6990, .T. ) ;
#19902=ADVANCED_FACE ( 'NONE', ( #2381 ), #13359, .T. ) ;
#19905=FACE_OUTER_BOUND ( 'NONE', #7555, .T. ) ;
#19909=EDGE_CURVE ( 'NONE', #19648, #19129, #14830, .T. ) ;
#19910=DIRECTION ( 'NONE',  ( 0.000000000000000000, -0.000000000000000000, 1.000000000000000000 ) ) ;
#19917=LINE ( 'NONE', #11942, #10683 ) ;
#19918=EDGE_LOOP ( 'NONE', ( #9275, #10972, #20358, #6743 ) ) ;
#19921=PLANE ( 'NONE',  #12444 ) ;
#19928=CARTESIAN_POINT ( 'NONE',  ( 0.000000000000000000, 9.000000000000001776, 0.000000000000000000 ) ) ;
#19937=ORIENTED_EDGE ( 'NONE', *, *, #3993, .T. ) ;
#19942=ADVANCED_FACE ( 'NONE', ( #19761 ), #2271, .F. ) ;
#19946=ORIENTED_EDGE ( 'NONE', *, *, #13605, .T. ) ;
#19948=CARTESIAN_POINT ( 'NONE',  ( -18.98630159782011262, 0.000000000000000000, 0.000000000000000000 ) ) ;
#19953=CARTESIAN_POINT ( 'NONE',  ( 0.000000000000000000, 9.000000000000001776, 1.000000000000000000 ) ) ;
#19962=CARTESIAN_POINT ( 'NONE',  ( 0.000000000000000000, 9.000000000000001776, 1.000000000000000000 ) ) ;
#19969=VERTEX_POINT ( 'NONE', #10128 ) ;
#19985=DIRECTION ( 'NONE',  ( -1.000000000000000000, 0.000000000000000000, 0.000000000000000000 ) ) ;
#19986=ORIENTED_EDGE ( 'NONE', *, *, #15869, .T. ) ;
#19987=ORIENTED_EDGE ( 'NONE', *, *, #664, .F. ) ;
#19989=CARTESIAN_POINT ( 'NONE',  ( 0.000000000000000000, 4.999999999999999112, 1.000000000000000000 ) ) ;
#19992=VECTOR ( 'NONE', #3320, 1000.000000000000000 ) ;
#19993=CARTESIAN_POINT ( 'NONE',  ( 15.86404127825609400, 9.000000000000001776, 0.000000000000000000 ) ) ;
#19994=DIRECTION ( 'NONE',  ( -0.000000000000000000, -0.000000000000000000, -1.000000000000000000 ) ) ;
#20006=ADVANCED_FACE ( 'NONE', ( #14360 ), #15731, .T. ) ;
#20007=VECTOR ( 'NONE', #10059, 1000.000000000000000 ) ;
#20008=LINE ( 'NONE', #5671, #3694 ) ;
#20012=ORIENTED_EDGE ( 'NONE', *, *, #1937, .T. ) ;
#20015=CARTESIAN_POINT ( 'NONE',  ( -0.1250000000000035805, 9.000000000000000000, 1.000000000000000000 ) ) ;
#20016=ORIENTED_EDGE ( 'NONE', *, *, #11829, .F. ) ;
#20017=EDGE_CURVE ( 'NONE', #16495, #7639, #18985, .T. ) ;
#20018=VERTEX_POINT ( 'NONE', #15831 ) ;
#20021=VECTOR ( 'NONE', #15632, 1000.000000000000000 ) ;
#20023=LINE ( 'NONE', #8722, #6577 ) ;
#20024=AXIS2_PLACEMENT_3D ( 'NONE', #20407, #13795, #5860 ) ;
#20025=LINE ( 'NONE', #10497, #6648 ) ;
#20028=DIRECTION ( 'NONE',  ( 0.000000000000000000, -0.000000000000000000, 1.000000000000000000 ) ) ;
#20030=EDGE_CURVE ( 'NONE', #8332, #17247, #4641, .T. ) ;
#20031=DIRECTION ( 'NONE',  ( 0.000000000000000000, -1.000000000000000000, 0.000000000000000000 ) ) ;
#20034=VECTOR ( 'NONE', #18683, 1000.000000000000000 ) ;
#20044=ORIENTED_EDGE ( 'NONE', *, *, #471, .F. ) ;
#20046=DIRECTION ( 'NONE',  ( 1.000000000000000000, 0.000000000000000000, 0.000000000000000000 ) ) ;
#20047=ORIENTED_EDGE ( 'NONE', *, *, #11235, .F. ) ;
#20053=CARTESIAN_POINT ( 'NONE',  ( 0.000000000000000000, 9.000000000000001776, 0.000000000000000000 ) ) ;
#20055=CARTESIAN_POINT ( 'NONE',  ( -17.05017143803810242, 4.999999999999999112, 0.000000000000000000 ) ) ;
#20058=ADVANCED_FACE ( 'NONE', ( #8968 ), #7413, .T. ) ;
#20062=PLANE ( 'NONE',  #18062 ) ;
#20064=LINE ( 'NONE', #12198, #4866 ) ;
#20070=ORIENTED_EDGE ( 'NONE', *, *, #1913, .F. ) ;
#20074=ORIENTED_EDGE ( 'NONE', *, *, #15603, .T. ) ;
#20091=DIRECTION ( 'NONE',  ( 0.000000000000000000, 1.000000000000000000, 0.000000000000000000 ) ) ;
#20092=DIRECTION ( 'NONE',  ( 1.000000000000000000, 0.000000000000000000, 0.000000000000000000 ) ) ;
#20099=PLANE ( 'NONE',  #1879 ) ;
#20102=DIRECTION ( 'NONE',  ( -0.000000000000000000, -0.000000000000000000, -1.000000000000000000 ) ) ;
#20103=FACE_OUTER_BOUND ( 'NONE', #14351, .T. ) ;
#20106=DIRECTION ( 'NONE',  ( 0.000000000000000000, 1.000000000000000000, 0.000000000000000000 ) ) ;
#20107=DIRECTION ( 'NONE',  ( -0.000000000000000000, 0.000000000000000000, -1.000000000000000000 ) ) ;
#20109=CARTESIAN_POINT ( 'NONE',  ( 0.000000000000000000, 4.999999999999999112, 0.000000000000000000 ) ) ;
#20113=ADVANCED_FACE ( 'NONE', ( #18597 ), #17608, .T. ) ;
#20122=ADVANCED_FACE ( 'NONE', ( #10643 ), #14249, .T. ) ;
#20123=DIRECTION ( 'NONE',  ( 0.000000000000000000, -0.000000000000000000, 1.000000000000000000 ) ) ;
#20131=VECTOR ( 'NONE', #8233, 1000.000000000000000 ) ;
#20137=CARTESIAN_POINT ( 'NONE',  ( 0.000000000000000000, 9.000000000000001776, 1.000000000000000000 ) ) ;
#20145=ORIENTED_EDGE ( 'NONE', *, *, #11498, .T. ) ;
#20149=ORIENTED_EDGE ( 'NONE', *, *, #12484, .F. ) ;
#20150=VECTOR ( 'NONE', #11823, 1000.000000000000000 ) ;
#20155=VERTEX_POINT ( 'NONE', #12691 ) ;
#20156=LINE ( 'NONE', #5817, #11524 ) ;
#20160=FACE_OUTER_BOUND ( 'NONE', #5117, .T. ) ;
#20166=ADVANCED_FACE ( 'NONE', ( #7989 ), #19197, .T. ) ;
#20176=CARTESIAN_POINT ( 'NONE',  ( 5.683390479346035029, 4.999999999999999112, 0.000000000000000000 ) ) ;
#20190=DIRECTION ( 'NONE',  ( -0.000000000000000000, -0.000000000000000000, -1.000000000000000000 ) ) ;
#20194=ORIENTED_EDGE ( 'NONE', *, *, #17412, .T. ) ;
#20204=ORIENTED_EDGE ( 'NONE', *, *, #17568, .T. ) ;
#20207=ORIENTED_EDGE ( 'NONE', *, *, #3993, .F. ) ;
#20214=CARTESIAN_POINT ( 'NONE',  ( 13.92791111847407848, 0.000000000000000000, 1.000000000000000000 ) ) ;
#20216=DIRECTION ( 'NONE',  ( 0.000000000000000000, 1.000000000000000000, 0.000000000000000000 ) ) ;
#20224=VERTEX_POINT ( 'NONE', #4952 ) ;
#20226=EDGE_CURVE ( 'NONE', #68, #9026, #1818, .T. ) ;
#20233=CARTESIAN_POINT ( 'NONE',  ( 26.79469207716614676, 9.000000000000001776, 1.000000000000000000 ) ) ;
#20234=LINE ( 'NONE', #12064, #1020 ) ;
#20240=ORIENTED_EDGE ( 'NONE', *, *, #2333, .T. ) ;
#20242=DIRECTION ( 'NONE',  ( 0.000000000000000000, 1.000000000000000000, 0.000000000000000000 ) ) ;
#20247=FACE_OUTER_BOUND ( 'NONE', #15736, .T. ) ;
#20251=VERTEX_POINT ( 'NONE', #14780 ) ;
#20255=EDGE_LOOP ( 'NONE', ( #18397, #10590, #605, #7861 ) ) ;
#20258=LINE ( 'NONE', #5918, #20034 ) ;
#20261=VECTOR ( 'NONE', #1613, 1000.000000000000000 ) ;
#20271=VERTEX_POINT ( 'NONE', #6934 ) ;
#20280=EDGE_CURVE ( 'NONE', #16495, #16469, #19299, .T. ) ;
#20286=PLANE ( 'NONE',  #17377 ) ;
#20290=EDGE_CURVE ( 'NONE', #10647, #16179, #8413, .T. ) ;
#20292=VERTEX_POINT ( 'NONE', #457 ) ;
#20297=LINE ( 'NONE', #12330, #17003 ) ;
#20299=ORIENTED_EDGE ( 'NONE', *, *, #13739, .T. ) ;
#20301=CARTESIAN_POINT ( 'NONE',  ( 21.67243175760212637, 9.000000000000001776, 1.000000000000000000 ) ) ;
#20303=LINE ( 'NONE', #5964, #114 ) ;
#20304=VERTEX_POINT ( 'NONE', #13301 ) ;
#20306=FACE_OUTER_BOUND ( 'NONE', #15832, .T. ) ;
#20315=LINE ( 'NONE', #14433, #8045 ) ;
#20317=VECTOR ( 'NONE', #4703, 1000.000000000000000 ) ;
#20320=VERTEX_POINT ( 'NONE', #8507 ) ;
#20324=VECTOR ( 'NONE', #19553, 1000.000000000000000 ) ;
#20326=DIRECTION ( 'NONE',  ( -0.000000000000000000, -0.000000000000000000, -1.000000000000000000 ) ) ;
#20331=CARTESIAN_POINT ( 'NONE',  ( 6.183390479346035917, 9.000000000000001776, 1.000000000000000000 ) ) ;
#20333=LINE ( 'NONE', #10816, #15375 ) ;
#20336=DIRECTION ( 'NONE',  ( 0.000000000000000000, 1.000000000000000000, 0.000000000000000000 ) ) ;
#20339=ORIENTED_EDGE ( 'NONE', *, *, #7457, .T. ) ;
#20341=LINE ( 'NONE', #18561, #17056 ) ;
#20346=DIRECTION ( 'NONE',  ( -0.000000000000000000, -0.000000000000000000, -1.000000000000000000 ) ) ;
#20347=CIRCLE ( 'NONE', #15983, 0.4999999999999987232 ) ;
#20348=ORIENTED_EDGE ( 'NONE', *, *, #20017, .T. ) ;
#20351=VECTOR ( 'NONE', #17004, 1000.000000000000000 ) ;
#20354=EDGE_CURVE ( 'NONE', #3944, #2453, #11439, .T. ) ;
#20358=ORIENTED_EDGE ( 'NONE', *, *, #6760, .T. ) ;
#20359=LINE ( 'NONE', #18375, #20701 ) ;
#20364=DIRECTION ( 'NONE',  ( 1.000000000000000000, 0.000000000000000000, 0.000000000000000000 ) ) ;
#20370=CARTESIAN_POINT ( 'NONE',  ( -3.999999999999999112, -7.500000000000047073, 9.999999999999998224 ) ) ;
#20380=LINE ( 'NONE', #6350, #15300 ) ;
#20381=EDGE_LOOP ( 'NONE', ( #1053, #6067, #8207, #8508 ) ) ;
#20385=EDGE_CURVE ( 'NONE', #12897, #9608, #15286, .T. ) ;
#20391=VECTOR ( 'NONE', #1623, 1000.000000000000000 ) ;
#20395=AXIS2_PLACEMENT_3D ( 'NONE', #12372, #10598, #20028 ) ;
#20400=ORIENTED_EDGE ( 'NONE', *, *, #12042, .T. ) ;
#20407=CARTESIAN_POINT ( 'NONE',  ( 13.50000000000000178, 7.806255641895631925E-15, 2.000000000000000000 ) ) ;
#20412=SURFACE_SIDE_STYLE ('',( #12337 ) ) ;
#20413=ORIENTED_EDGE ( 'NONE', *, *, #4749, .T. ) ;
#20415=VERTEX_POINT ( 'NONE', #5784 ) ;
#20422=VECTOR ( 'NONE', #20346, 1000.000000000000000 ) ;
#20431=DIRECTION ( 'NONE',  ( 1.000000000000000000, 0.000000000000000000, 0.000000000000000000 ) ) ;
#20435=ORIENTED_EDGE ( 'NONE', *, *, #4630, .F. ) ;
#20439=ORIENTED_EDGE ( 'NONE', *, *, #9585, .F. ) ;
#20442=DIRECTION ( 'NONE',  ( -0.000000000000000000, -0.000000000000000000, -1.000000000000000000 ) ) ;
#20450=DIRECTION ( 'NONE',  ( 0.000000000000000000, 1.000000000000000000, 0.000000000000000000 ) ) ;
#20456=LINE ( 'NONE', #4333, #13053 ) ;
#20461=LINE ( 'NONE', #13844, #367 ) ;
#20465=EDGE_LOOP ( 'NONE', ( #18954, #18759, #3134, #324 ) ) ;
#20470=VERTEX_POINT ( 'NONE', #20015 ) ;
#20472=EDGE_CURVE ( 'NONE', #3752, #1149, #15189, .T. ) ;
#20474=DIRECTION ( 'NONE',  ( 0.000000000000000000, 1.000000000000000000, 0.000000000000000000 ) ) ;
#20478=FACE_OUTER_BOUND ( 'NONE', #10566, .T. ) ;
#20480=DIRECTION ( 'NONE',  ( -1.000000000000000000, 0.000000000000000000, 0.000000000000000000 ) ) ;
#20484=VECTOR ( 'NONE', #9772, 1000.000000000000000 ) ;
#20486=ORIENTED_EDGE ( 'NONE', *, *, #4892, .T. ) ;
#20489=ADVANCED_FACE ( 'NONE', ( #2636 ), #18446, .T. ) ;
#20491=PLANE ( 'NONE',  #14976 ) ;
#20494=ORIENTED_EDGE ( 'NONE', *, *, #2905, .T. ) ;
#20497=FACE_OUTER_BOUND ( 'NONE', #1228, .T. ) ;
#20498=EDGE_CURVE ( 'NONE', #7526, #8019, #19917, .T. ) ;
#20501=LINE ( 'NONE', #14092, #12032 ) ;
#20512=ORIENTED_EDGE ( 'NONE', *, *, #5809, .T. ) ;
#20514=DIRECTION ( 'NONE',  ( 1.000000000000000000, 0.000000000000000000, 0.000000000000000000 ) ) ;
#20530=DIRECTION ( 'NONE',  ( 0.000000000000000000, 1.000000000000000000, -0.000000000000000000 ) ) ;
#20540=ORIENTED_EDGE ( 'NONE', *, *, #4200, .T. ) ;
#20547=ADVANCED_FACE ( 'NONE', ( #7557 ), #7863, .T. ) ;
#20550=DIRECTION ( 'NONE',  ( -0.000000000000000000, -0.000000000000000000, -1.000000000000000000 ) ) ;
#20562=DIRECTION ( 'NONE',  ( 1.000000000000000000, 0.000000000000000000, -0.000000000000000000 ) ) ;
#20565=ORIENTED_EDGE ( 'NONE', *, *, #4912, .F. ) ;
#20566=CARTESIAN_POINT ( 'NONE',  ( 0.000000000000000000, 4.999999999999999112, 0.000000000000000000 ) ) ;
#20568=CARTESIAN_POINT ( 'NONE',  ( -13.97248077590530180, -0.1818351014256275322, 0.8937704884164922037 ) ) ;
#20574=DIRECTION ( 'NONE',  ( -0.000000000000000000, -0.000000000000000000, -1.000000000000000000 ) ) ;
#20575=CARTESIAN_POINT ( 'NONE',  ( -1.561130159782011306, 0.000000000000000000, 1.000000000000000000 ) ) ;
#20577=DIRECTION ( 'NONE',  ( -1.000000000000000000, 0.000000000000000000, 0.000000000000000000 ) ) ;
#20582=ADVANCED_FACE ( 'NONE', ( #6096 ), #12660, .T. ) ;
#20587=ORIENTED_EDGE ( 'NONE', *, *, #10257, .T. ) ;
#20592=ORIENTED_EDGE ( 'NONE', *, *, #4302, .F. ) ;
#20597=CARTESIAN_POINT ( 'NONE',  ( 0.3749999999999968914, 9.000000000000000000, 0.000000000000000000 ) ) ;
#20598=LINE ( 'NONE', #8810, #11300 ) ;
#20607=AXIS2_PLACEMENT_3D ( 'NONE', #13467, #4239, #9057 ) ;
#20620=CARTESIAN_POINT ( 'NONE',  ( 0.000000000000000000, 4.999999999999999112, 0.000000000000000000 ) ) ;
#20626=DIRECTION ( 'NONE',  ( -0.000000000000000000, 0.000000000000000000, 1.000000000000000000 ) ) ;
#20628=EDGE_CURVE ( 'NONE', #17249, #16180, #8078, .T. ) ;
#20636=ORIENTED_EDGE ( 'NONE', *, *, #19634, .F. ) ;
#20638=DIRECTION ( 'NONE',  ( 0.000000000000000000, -0.000000000000000000, 1.000000000000000000 ) ) ;
#20642=CARTESIAN_POINT ( 'NONE',  ( 0.000000000000000000, 9.000000000000001776, 1.000000000000000000 ) ) ;
#20650=DIRECTION ( 'NONE',  ( 1.000000000000000000, 0.000000000000000000, 0.000000000000000000 ) ) ;
#20652=EDGE_CURVE ( 'NONE', #14572, #6961, #4927, .T. ) ;
#20662=PLANE ( 'NONE',  #8439 ) ;
#20664=VECTOR ( 'NONE', #593, 1000.000000000000000 ) ;
#20667=LINE ( 'NONE', #11521, #14686 ) ;
#20670=CARTESIAN_POINT ( 'NONE',  ( -1.561130159782011306, 0.000000000000000000, 1.000000000000000000 ) ) ;
#20672=LINE ( 'NONE', #9569, #17700 ) ;
#20674=PLANE ( 'NONE',  #9387 ) ;
#20682=AXIS2_PLACEMENT_3D ( 'NONE', #14992, #370, #3812 ) ;
#20689=VERTEX_POINT ( 'NONE', #3669 ) ;
#20690=PLANE ( 'NONE',  #14771 ) ;
#20696=CARTESIAN_POINT ( 'NONE',  ( -2.061130159782011972, 4.999999999999999112, 1.000000000000000000 ) ) ;
#20699=DIRECTION ( 'NONE',  ( 0.000000000000000000, 1.000000000000000000, -0.000000000000000000 ) ) ;
#20701=VECTOR ( 'NONE', #16995, 1000.000000000000000 ) ;
#20703=FILL_AREA_STYLE_COLOUR ( '', #4854 ) ;
#20705=VERTEX_POINT ( 'NONE', #3464 ) ;
#20708=CARTESIAN_POINT ( 'NONE',  ( 0.000000000000000000, 9.000000000000001776, 1.000000000000000000 ) ) ;
#20717=EDGE_LOOP ( 'NONE', ( #4452, #6608, #14516, #15139 ) ) ;
ENDSEC;
END-ISO-10303-21;
